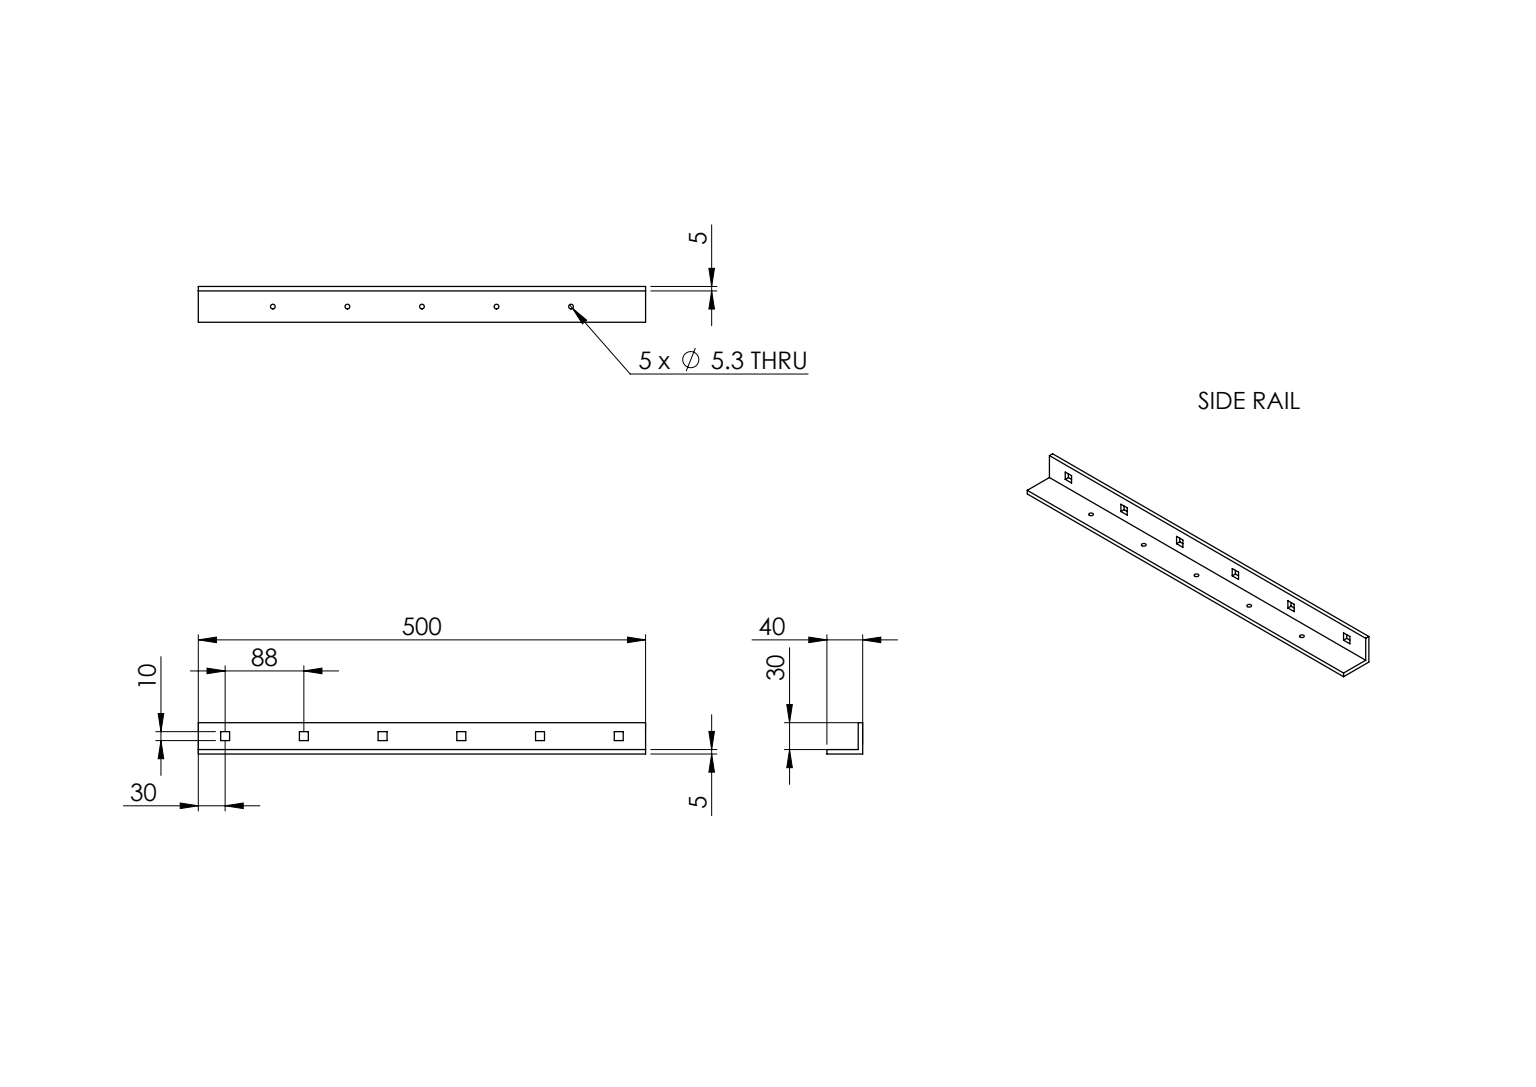
ISO-10303-21;
HEADER;
FILE_DESCRIPTION (('STEP AP214'),
    '1' );
FILE_NAME ('side rail.step',
    '2026-10-24T11:01:53',
    ( '' ),
    ( '' ),
    'SwSTEP 2.0',
    'SolidWorks 2026',
    '' );
FILE_SCHEMA (( 'AUTOMOTIVE_DESIGN' ));
ENDSEC;

DATA;
#13=PRODUCT_DEFINITION_FORMATION_WITH_SPECIFIED_SOURCE ( 'ANY', '', #8583, .NOT_KNOWN. ) ;
#18=CARTESIAN_POINT ( 'NONE',  ( 386.6666666666666288, -15.00000000000000000, 165.1500000000000625 ) ) ;
#24=VERTEX_POINT ( 'NONE', #6412 ) ;
#26=CARTESIAN_POINT ( 'NONE',  ( -30.00000000000000000, 15.00000000000000000, 145.0000000000000284 ) ) ;
#31=CARTESIAN_POINT ( 'NONE',  ( -4.999999999999998224, -4.999999999999998224, 145.0000000000000284 ) ) ;
#46=AXIS2_PLACEMENT_3D ( 'NONE', #70, #7390, #6602 ) ;
#48=VECTOR ( 'NONE', #1988, 1000.000000000000000 ) ;
#54=VERTEX_POINT ( 'NONE', #1769 ) ;
#58=VERTEX_POINT ( 'NONE', #5981 ) ;
#60=EDGE_CURVE ( 'NONE', #24, #4191, #63, .T. ) ;
#63=LINE ( 'NONE', #5464, #2595 ) ;
#67=EDGE_CURVE ( 'NONE', #3923, #3144, #6728, .T. ) ;
#70=CARTESIAN_POINT ( 'NONE',  ( 219.9999999999999716, -14.99999999999999822, 162.5000000000000853 ) ) ;
#87=ADVANCED_FACE ( 'NONE', ( #7344 ), #1423, .F. ) ;
#111=AXIS2_PLACEMENT_3D ( 'NONE', #1042, #3694, #1743 ) ;
#117=ORIENTED_EDGE ( 'NONE', *, *, #2503, .F. ) ;
#124=ORIENTED_EDGE ( 'NONE', *, *, #3492, .T. ) ;
#125=LINE ( 'NONE', #5958, #4603 ) ;
#149=CARTESIAN_POINT ( 'NONE',  ( -30.00000000000002842, -15.00000000000000000, 180.0000000000000284 ) ) ;
#156=VECTOR ( 'NONE', #5813, 1000.000000000000000 ) ;
#162=DIRECTION ( 'NONE',  ( -0.000000000000000000, -0.000000000000000000, 1.000000000000000000 ) ) ;
#167=ADVANCED_FACE ( 'NONE', ( #3513 ), #4000, .F. ) ;
#169=EDGE_LOOP ( 'NONE', ( #5952, #1913, #7757, #4086 ) ) ;
#170=DIRECTION ( 'NONE',  ( -1.000000000000000000, 0.000000000000000000, -0.000000000000000000 ) ) ;
#174=DIRECTION ( 'NONE',  ( 0.000000000000000000, -1.000000000000000000, 0.000000000000000000 ) ) ;
#182=CARTESIAN_POINT ( 'NONE',  ( 269.0000000000000000, -4.999999999999998224, 145.0000000000000284 ) ) ;
#186=VERTEX_POINT ( 'NONE', #5337 ) ;
#190=ORIENTED_EDGE ( 'NONE', *, *, #4626, .T. ) ;
#201=EDGE_CURVE ( 'NONE', #7722, #4892, #6771, .T. ) ;
#202=EDGE_CURVE ( 'NONE', #3923, #6024, #3423, .T. ) ;
#203=LINE ( 'NONE', #2266, #5375 ) ;
#208=ORIENTED_EDGE ( 'NONE', *, *, #6764, .T. ) ;
#220=AXIS2_PLACEMENT_3D ( 'NONE', #6944, #7654, #6292 ) ;
#234=EDGE_CURVE ( 'NONE', #3505, #4164, #2178, .T. ) ;
#238=VERTEX_POINT ( 'NONE', #4948 ) ;
#241=DIRECTION ( 'NONE',  ( 0.000000000000000000, 0.000000000000000000, 1.000000000000000000 ) ) ;
#244=FACE_OUTER_BOUND ( 'NONE', #4831, .T. ) ;
#245=LINE ( 'NONE', #4910, #2842 ) ;
#249=EDGE_CURVE ( 'NONE', #7704, #6568, #408, .T. ) ;
#254=ORIENTED_EDGE ( 'NONE', *, *, #6075, .T. ) ;
#255=DIRECTION ( 'NONE',  ( 0.000000000000000000, -1.000000000000000000, 0.000000000000000000 ) ) ;
#259=DIRECTION ( 'NONE',  ( 0.000000000000000000, 0.000000000000000000, 1.000000000000000000 ) ) ;
#263=VECTOR ( 'NONE', #6923, 1000.000000000000000 ) ;
#287=PLANE ( 'NONE',  #7700 ) ;
#289=CARTESIAN_POINT ( 'NONE',  ( 219.9999999999999716, -20.00000000000000000, 165.1500000000000625 ) ) ;
#298=DIRECTION ( 'NONE',  ( 0.000000000000000000, 0.000000000000000000, 1.000000000000000000 ) ) ;
#309=DIRECTION ( 'NONE',  ( 0.000000000000000000, 0.000000000000000000, 1.000000000000000000 ) ) ;
#318=ORIENTED_EDGE ( 'NONE', *, *, #3170, .T. ) ;
#324=DIRECTION ( 'NONE',  ( -0.000000000000000000, -0.000000000000000000, -1.000000000000000000 ) ) ;
#331=AXIS2_PLACEMENT_3D ( 'NONE', #650, #3395, #2654 ) ;
#333=CARTESIAN_POINT ( 'NONE',  ( 170.9999999999999716, 5.000000000000001776, 140.0000000000000000 ) ) ;
#347=ORIENTED_EDGE ( 'NONE', *, *, #4193, .T. ) ;
#361=ADVANCED_FACE ( 'NONE', ( #4903 ), #2861, .F. ) ;
#363=EDGE_CURVE ( 'NONE', #6062, #5755, #7748, .T. ) ;
#375=ORIENTED_EDGE ( 'NONE', *, *, #4660, .F. ) ;
#386=ORIENTED_EDGE ( 'NONE', *, *, #234, .T. ) ;
#388=LINE ( 'NONE', #2410, #2981 ) ;
#406=AXIS2_PLACEMENT_3D ( 'NONE', #5690, #1942, #2315 ) ;
#407=ORIENTED_EDGE ( 'NONE', *, *, #3455, .T. ) ;
#408=LINE ( 'NONE', #3556, #5504 ) ;
#413=ORIENTED_EDGE ( 'NONE', *, *, #6908, .F. ) ;
#416=SURFACE_STYLE_FILL_AREA ( #6943 ) ;
#427=CARTESIAN_POINT ( 'NONE',  ( 357.0000000000000000, -4.999999999999998224, 145.0000000000000284 ) ) ;
#429=ORIENTED_EDGE ( 'NONE', *, *, #1847, .T. ) ;
#431=DIRECTION ( 'NONE',  ( -1.734723475976807341E-16, 1.000000000000000000, 0.000000000000000000 ) ) ;
#433=DIRECTION ( 'NONE',  ( 0.000000000000000000, 0.000000000000000000, 1.000000000000000000 ) ) ;
#445=EDGE_CURVE ( 'NONE', #1439, #7609, #7238, .T. ) ;
#446=DIRECTION ( 'NONE',  ( 0.000000000000000000, 0.000000000000000000, 1.000000000000000000 ) ) ;
#448=ORIENTED_EDGE ( 'NONE', *, *, #1374, .T. ) ;
#464=DIRECTION ( 'NONE',  ( 0.000000000000000000, 0.000000000000000000, 1.000000000000000000 ) ) ;
#466=EDGE_LOOP ( 'NONE', ( #1944, #2418, #2156, #4919 ) ) ;
#472=APPLICATION_CONTEXT ( 'automotive_design' ) ;
#473=CARTESIAN_POINT ( 'NONE',  ( -30.00000000000002842, -20.00000000000000000, 180.0000000000000284 ) ) ;
#495=CARTESIAN_POINT ( 'NONE',  ( 136.6666666666666288, -14.99999999999999822, 162.5000000000000853 ) ) ;
#503=AXIS2_PLACEMENT_3D ( 'NONE', #3389, #7471, #6027 ) ;
#516=CIRCLE ( 'NONE', #3995, 2.649999999999985700 ) ;
#517=VECTOR ( 'NONE', #7391, 1000.000000000000000 ) ;
#522=CARTESIAN_POINT ( 'NONE',  ( 444.9999999999999432, -4.999999999999998224, 139.9990000000000236 ) ) ;
#524=CYLINDRICAL_SURFACE ( 'NONE', #783, 2.649999999999985700 ) ;
#527=ORIENTED_EDGE ( 'NONE', *, *, #5024, .F. ) ;
#539=AXIS2_PLACEMENT_3D ( 'NONE', #8100, #4108, #804 ) ;
#540=FACE_OUTER_BOUND ( 'NONE', #466, .T. ) ;
#545=CARTESIAN_POINT ( 'NONE',  ( 347.0000000000000000, 5.000000000000001776, 145.0000000000000284 ) ) ;
#547=DIRECTION ( 'NONE',  ( 0.000000000000000000, -1.000000000000000000, 0.000000000000000000 ) ) ;
#551=EDGE_CURVE ( 'NONE', #2756, #4735, #3107, .T. ) ;
#553=CARTESIAN_POINT ( 'NONE',  ( 259.0000000000000000, -4.999999999999998224, 140.0000000000000000 ) ) ;
#575=CARTESIAN_POINT ( 'NONE',  ( -30.00000000000002842, -20.00000000000000000, 180.0000000000000284 ) ) ;
#578=EDGE_CURVE ( 'NONE', #4191, #4735, #5829, .T. ) ;
#580=EDGE_CURVE ( 'NONE', #8517, #6781, #7849, .T. ) ;
#581=STYLED_ITEM('',(#8650),#4654);
#592=AXIS2_PLACEMENT_3D ( 'NONE', #1582, #4234, #309 ) ;
#594=AXIS2_PLACEMENT_3D ( 'NONE', #3123, #464, #5764 ) ;
#601=FACE_BOUND ( 'NONE', #6016, .T. ) ;
#603=VECTOR ( 'NONE', #2035, 1000.000000000000000 ) ;
#604=ORIENTED_EDGE ( 'NONE', *, *, #7855, .F. ) ;
#606=FACE_OUTER_BOUND ( 'NONE', #8585, .T. ) ;
#609=FACE_OUTER_BOUND ( 'NONE', #8309, .T. ) ;
#610=DIRECTION ( 'NONE',  ( 0.000000000000000000, -1.000000000000000000, 0.000000000000000000 ) ) ;
#611=ORIENTED_EDGE ( 'NONE', *, *, #6429, .F. ) ;
#616=VECTOR ( 'NONE', #2532, 1000.000000000000000 ) ;
#640=ORIENTED_EDGE ( 'NONE', *, *, #7790, .T. ) ;
#641=CARTESIAN_POINT ( 'NONE',  ( 444.9999999999999432, 5.000000000000000000, 145.0000000000000284 ) ) ;
#650=CARTESIAN_POINT ( 'NONE',  ( 82.99999999999998579, -4.999999999999998224, 139.9990000000000236 ) ) ;
#655=FACE_OUTER_BOUND ( 'NONE', #4653, .T. ) ;
#656=EDGE_LOOP ( 'NONE', ( #7632, #980, #7793, #6433 ) ) ;
#662=DIRECTION ( 'NONE',  ( -0.000000000000000000, 1.000000000000000000, -0.000000000000000000 ) ) ;
#667=CARTESIAN_POINT ( 'NONE',  ( 434.9999999999999432, 5.000000000000001776, 140.0000000000000000 ) ) ;
#673=DIRECTION ( 'NONE',  ( -0.000000000000000000, -0.000000000000000000, 1.000000000000000000 ) ) ;
#675=ORIENTED_EDGE ( 'NONE', *, *, #4538, .T. ) ;
#679=CARTESIAN_POINT ( 'NONE',  ( 386.6666666666666288, -20.00000000000000000, 159.8500000000001080 ) ) ;
#680=LINE ( 'NONE', #6020, #603 ) ;
#681=EDGE_CURVE ( 'NONE', #54, #5626, #751, .T. ) ;
#691=CARTESIAN_POINT ( 'NONE',  ( 259.0000000000000000, -4.999999999999998224, 145.0000000000000284 ) ) ;
#692=DIRECTION ( 'NONE',  ( 0.000000000000000000, 0.000000000000000000, 1.000000000000000000 ) ) ;
#694=DIRECTION ( 'NONE',  ( 1.000000000000000000, 1.734723475976807587E-16, 0.000000000000000000 ) ) ;
#698=ORIENTED_EDGE ( 'NONE', *, *, #7696, .T. ) ;
#705=DIRECTION ( 'NONE',  ( 1.000000000000000000, 0.000000000000000000, 0.000000000000000000 ) ) ;
#706=EDGE_CURVE ( 'NONE', #6409, #7056, #2096, .T. ) ;
#715=EDGE_LOOP ( 'NONE', ( #5309, #6953, #3557, #6643 ) ) ;
#716=VERTEX_POINT ( 'NONE', #3406 ) ;
#722=EDGE_LOOP ( 'NONE', ( #7433, #7623, #8054, #2319 ) ) ;
#729=DIRECTION ( 'NONE',  ( -0.000000000000000000, 1.000000000000000000, -0.000000000000000000 ) ) ;
#730=VERTEX_POINT ( 'NONE', #3974 ) ;
#733=DIRECTION ( 'NONE',  ( 0.000000000000000000, -1.000000000000000000, 0.000000000000000000 ) ) ;
#734=DIRECTION ( 'NONE',  ( 1.000000000000000000, 1.734723475976807587E-16, 0.000000000000000000 ) ) ;
#740=VECTOR ( 'NONE', #3211, 1000.000000000000000 ) ;
#749=VECTOR ( 'NONE', #5021, 1000.000000000000000 ) ;
#751=LINE ( 'NONE', #3447, #4670 ) ;
#753=ADVANCED_FACE ( 'NONE', ( #4656 ), #3358, .F. ) ;
#763=CARTESIAN_POINT ( 'NONE',  ( -30.00000000000000000, 15.00000000000000000, 145.0000000000000284 ) ) ;
#780=CARTESIAN_POINT ( 'NONE',  ( 434.9999999999999432, -4.999999999999998224, 145.0000000000000284 ) ) ;
#783=AXIS2_PLACEMENT_3D ( 'NONE', #5091, #5820, #5173 ) ;
#785=DIRECTION ( 'NONE',  ( 0.000000000000000000, 1.000000000000000000, 0.000000000000000000 ) ) ;
#786=ORIENTED_EDGE ( 'NONE', *, *, #578, .T. ) ;
#796=DIRECTION ( 'NONE',  ( -1.000000000000000000, 0.000000000000000000, 0.000000000000000000 ) ) ;
#804=DIRECTION ( 'NONE',  ( 0.000000000000000000, 0.000000000000000000, 1.000000000000000000 ) ) ;
#809=DIRECTION ( 'NONE',  ( 0.000000000000000000, 0.000000000000000000, 1.000000000000000000 ) ) ;
#819=VERTEX_POINT ( 'NONE', #4271 ) ;
#837=CARTESIAN_POINT ( 'NONE',  ( 347.0000000000000000, -4.999999999999998224, 145.0000000000000284 ) ) ;
#841=EDGE_CURVE ( 'NONE', #58, #2735, #4314, .T. ) ;
#849=EDGE_CURVE ( 'NONE', #874, #3144, #1486, .T. ) ;
#855=ORIENTED_EDGE ( 'NONE', *, *, #4193, .F. ) ;
#859=DIRECTION ( 'NONE',  ( -0.000000000000000000, 1.000000000000000000, -0.000000000000000000 ) ) ;
#861=ORIENTED_EDGE ( 'NONE', *, *, #3272, .T. ) ;
#874=VERTEX_POINT ( 'NONE', #6131 ) ;
#877=FACE_OUTER_BOUND ( 'NONE', #3003, .T. ) ;
#898=VECTOR ( 'NONE', #7582, 1000.000000000000000 ) ;
#902=DIRECTION ( 'NONE',  ( 0.000000000000000000, -0.000000000000000000, -1.000000000000000000 ) ) ;
#905=DIRECTION ( 'NONE',  ( 0.000000000000000000, 0.000000000000000000, -1.000000000000000000 ) ) ;
#911=FACE_OUTER_BOUND ( 'NONE', #8041, .T. ) ;
#920=CARTESIAN_POINT ( 'NONE',  ( 347.0000000000000000, -4.999999999999998224, 139.9990000000000236 ) ) ;
#925=FACE_BOUND ( 'NONE', #8290, .T. ) ;
#928=CARTESIAN_POINT ( 'NONE',  ( 470.0000000000000000, 15.00000000000000000, 140.0000000000000000 ) ) ;
#951=VERTEX_POINT ( 'NONE', #3223 ) ;
#955=LINE ( 'NONE', #3606, #3821 ) ;
#957=CARTESIAN_POINT ( 'NONE',  ( 219.9999999999999716, -20.00000000000000000, 162.5000000000000853 ) ) ;
#968=LINE ( 'NONE', #7447, #1506 ) ;
#970=PLANE ( 'NONE',  #4855 ) ;
#972=CARTESIAN_POINT ( 'NONE',  ( -30.00000000000002842, -20.00000000000000000, 180.0000000000000284 ) ) ;
#978=DIRECTION ( 'NONE',  ( 0.000000000000000000, 1.000000000000000000, 0.000000000000000000 ) ) ;
#979=ORIENTED_EDGE ( 'NONE', *, *, #3323, .F. ) ;
#980=ORIENTED_EDGE ( 'NONE', *, *, #7467, .T. ) ;
#984=ADVANCED_FACE ( 'NONE', ( #1052 ), #524, .F. ) ;
#986=ADVANCED_FACE ( 'NONE', ( #8495 ), #7673, .F. ) ;
#991=ORIENTED_EDGE ( 'NONE', *, *, #2182, .F. ) ;
#993=DIRECTION ( 'NONE',  ( -1.000000000000000000, 0.000000000000000000, 0.000000000000000000 ) ) ;
#1010=ADVANCED_FACE ( 'NONE', ( #6523 ), #8539, .F. ) ;
#1014=CARTESIAN_POINT ( 'NONE',  ( -4.999999999999998224, 5.000000000000001776, 139.9990000000000236 ) ) ;
#1023=ORIENTED_EDGE ( 'NONE', *, *, #5149, .T. ) ;
#1042=CARTESIAN_POINT ( 'NONE',  ( 386.6666666666666288, -15.00000000000000000, 162.5000000000000853 ) ) ;
#1048=ADVANCED_FACE ( 'NONE', ( #8418 ), #2454, .F. ) ;
#1050=DIRECTION ( 'NONE',  ( 0.000000000000000000, 0.000000000000000000, 1.000000000000000000 ) ) ;
#1052=FACE_OUTER_BOUND ( 'NONE', #5062, .T. ) ;
#1054=ORIENTED_EDGE ( 'NONE', *, *, #7248, .T. ) ;
#1055=DIRECTION ( 'NONE',  ( -1.000000000000000000, 0.000000000000000000, 0.000000000000000000 ) ) ;
#1067=LINE ( 'NONE', #8387, #5879 ) ;
#1078=ORIENTED_EDGE ( 'NONE', *, *, #5149, .F. ) ;
#1084=CARTESIAN_POINT ( 'NONE',  ( 347.0000000000000000, 5.000000000000001776, 145.0000000000000284 ) ) ;
#1092=CARTESIAN_POINT ( 'NONE',  ( -4.999999999999998224, 5.000000000000001776, 145.0000000000000284 ) ) ;
#1120=AXIS2_PLACEMENT_3D ( 'NONE', #2318, #4961, #4307 ) ;
#1123=VERTEX_POINT ( 'NONE', #2089 ) ;
#1125=DIRECTION ( 'NONE',  ( 1.000000000000000000, 0.000000000000000000, 0.000000000000000000 ) ) ;
#1126=FACE_OUTER_BOUND ( 'NONE', #2316, .T. ) ;
#1127=ORIENTED_EDGE ( 'NONE', *, *, #3594, .F. ) ;
#1129=ADVANCED_FACE ( 'NONE', ( #609 ), #3265, .F. ) ;
#1145=CARTESIAN_POINT ( 'NONE',  ( 269.0000000000000000, -4.999999999999998224, 145.0000000000000284 ) ) ;
#1149=EDGE_CURVE ( 'NONE', #3461, #2983, #5389, .T. ) ;
#1152=ADVANCED_FACE ( 'NONE', ( #3482 ), #8277, .T. ) ;
#1153=VECTOR ( 'NONE', #1857, 1000.000000000000000 ) ;
#1185=ORIENTED_EDGE ( 'NONE', *, *, #201, .F. ) ;
#1192=DIRECTION ( 'NONE',  ( 0.000000000000000000, 1.000000000000000000, 0.000000000000000000 ) ) ;
#1195=AXIS2_PLACEMENT_3D ( 'NONE', #7262, #694, #2743 ) ;
#1203=AXIS2_PLACEMENT_3D ( 'NONE', #5420, #8139, #5288 ) ;
#1204=ORIENTED_EDGE ( 'NONE', *, *, #4975, .T. ) ;
#1208=FACE_OUTER_BOUND ( 'NONE', #8313, .T. ) ;
#1210=CARTESIAN_POINT ( 'NONE',  ( 434.9999999999999432, -4.999999999999998224, 139.9990000000000236 ) ) ;
#1212=DIRECTION ( 'NONE',  ( -1.000000000000000000, 1.734723475976807341E-16, -0.000000000000000000 ) ) ;
#1213=EDGE_CURVE ( 'NONE', #730, #716, #6215, .T. ) ;
#1223=VECTOR ( 'NONE', #3407, 1000.000000000000000 ) ;
#1228=DIRECTION ( 'NONE',  ( -0.000000000000000000, 1.000000000000000000, -0.000000000000000000 ) ) ;
#1236=LINE ( 'NONE', #1279, #1910 ) ;
#1244=EDGE_CURVE ( 'NONE', #238, #4249, #5603, .T. ) ;
#1248=VERTEX_POINT ( 'NONE', #6169 ) ;
#1257=DIRECTION ( 'NONE',  ( 0.000000000000000000, -0.000000000000000000, -1.000000000000000000 ) ) ;
#1263=EDGE_CURVE ( 'NONE', #1874, #8118, #8146, .T. ) ;
#1276=EDGE_CURVE ( 'NONE', #2983, #951, #203, .T. ) ;
#1279=CARTESIAN_POINT ( 'NONE',  ( 82.99999999999998579, -4.999999999999998224, 145.0000000000000284 ) ) ;
#1281=VECTOR ( 'NONE', #1939, 1000.000000000000000 ) ;
#1286=CARTESIAN_POINT ( 'NONE',  ( 219.9999999999999716, -14.99999999999999822, 159.8500000000001080 ) ) ;
#1294=CARTESIAN_POINT ( 'NONE',  ( 0.000000000000000000, 0.000000000000000000, 145.0000000000000284 ) ) ;
#1313=CARTESIAN_POINT ( 'NONE',  ( 259.0000000000000000, -4.999999999999998224, 145.0000000000000284 ) ) ;
#1316=CARTESIAN_POINT ( 'NONE',  ( 181.0000000000000000, 5.000000000000000000, 145.0000000000000284 ) ) ;
#1318=LINE ( 'NONE', #1360, #3234 ) ;
#1320=CARTESIAN_POINT ( 'NONE',  ( 303.3333333333333144, -20.00000000000000000, 162.5000000000000853 ) ) ;
#1331=ORIENTED_EDGE ( 'NONE', *, *, #6988, .T. ) ;
#1335=CARTESIAN_POINT ( 'NONE',  ( 219.9999999999999716, -15.00000000000000000, 162.5000000000000853 ) ) ;
#1340=PLANE ( 'NONE',  #6168 ) ;
#1341=ADVANCED_FACE ( 'NONE', ( #1126 ), #3869, .F. ) ;
#1360=CARTESIAN_POINT ( 'NONE',  ( 444.9999999999999432, -4.999999999999998224, 140.0000000000000000 ) ) ;
#1362=CARTESIAN_POINT ( 'NONE',  ( 82.99999999999998579, -4.999999999999998224, 140.0000000000000000 ) ) ;
#1363=LINE ( 'NONE', #3985, #3019 ) ;
#1374=EDGE_CURVE ( 'NONE', #1123, #951, #3693, .T. ) ;
#1375=EDGE_CURVE ( 'NONE', #4726, #7555, #7127, .T. ) ;
#1377=DIRECTION ( 'NONE',  ( 1.000000000000000000, 0.000000000000000000, 0.000000000000000000 ) ) ;
#1386=ORIENTED_EDGE ( 'NONE', *, *, #1213, .T. ) ;
#1390=DIRECTION ( 'NONE',  ( 1.734723475976807587E-16, 1.000000000000000000, 0.000000000000000000 ) ) ;
#1406=CARTESIAN_POINT ( 'NONE',  ( 470.0000000000000000, 15.00000000000000000, 140.0000000000000000 ) ) ;
#1413=CARTESIAN_POINT ( 'NONE',  ( 434.9999999999999432, 5.000000000000001776, 139.9990000000000236 ) ) ;
#1421=ORIENTED_EDGE ( 'NONE', *, *, #7067, .T. ) ;
#1423=PLANE ( 'NONE',  #5781 ) ;
#1427=VECTOR ( 'NONE', #7633, 1000.000000000000000 ) ;
#1436=ORIENTED_EDGE ( 'NONE', *, *, #4897, .F. ) ;
#1439=VERTEX_POINT ( 'NONE', #2688 ) ;
#1441=CARTESIAN_POINT ( 'NONE',  ( 170.9999999999999716, 5.000000000000001776, 145.0000000000000284 ) ) ;
#1442=AXIS2_PLACEMENT_3D ( 'NONE', #2110, #4768, #809 ) ;
#1445=FACE_OUTER_BOUND ( 'NONE', #6630, .T. ) ;
#1449=LINE ( 'NONE', #4887, #2264 ) ;
#1456=EDGE_CURVE ( 'NONE', #7186, #4028, #5849, .T. ) ;
#1465=DIRECTION ( 'NONE',  ( -1.000000000000000000, 0.000000000000000000, 0.000000000000000000 ) ) ;
#1466=DIRECTION ( 'NONE',  ( 0.000000000000000000, -1.000000000000000000, 0.000000000000000000 ) ) ;
#1472=CARTESIAN_POINT ( 'NONE',  ( 434.9999999999999432, -4.999999999999998224, 140.0000000000000000 ) ) ;
#1475=ORIENTED_EDGE ( 'NONE', *, *, #3348, .T. ) ;
#1486=CIRCLE ( 'NONE', #7458, 2.649999999999985700 ) ;
#1492=CARTESIAN_POINT ( 'NONE',  ( 0.000000000000000000, 0.000000000000000000, 140.0000000000000000 ) ) ;
#1506=VECTOR ( 'NONE', #6180, 1000.000000000000000 ) ;
#1507=ORIENTED_EDGE ( 'NONE', *, *, #6503, .T. ) ;
#1519=DIRECTION ( 'NONE',  ( 0.000000000000000000, 1.000000000000000000, 0.000000000000000000 ) ) ;
#1520=CARTESIAN_POINT ( 'NONE',  ( -30.00000000000000000, 15.00000000000000000, 145.0000000000000284 ) ) ;
#1531=CARTESIAN_POINT ( 'NONE',  ( 5.000000000000001776, -4.999999999999998224, 145.0000000000000284 ) ) ;
#1534=ORIENTED_EDGE ( 'NONE', *, *, #3805, .T. ) ;
#1545=ORIENTED_EDGE ( 'NONE', *, *, #5785, .T. ) ;
#1547=CARTESIAN_POINT ( 'NONE',  ( 470.0000000000000000, -20.00000000000000000, 180.0000000000000284 ) ) ;
#1549=VERTEX_POINT ( 'NONE', #5244 ) ;
#1559=CARTESIAN_POINT ( 'NONE',  ( 470.0000000000000000, 15.00000000000000000, 145.0000000000000284 ) ) ;
#1571=CARTESIAN_POINT ( 'NONE',  ( 357.0000000000000000, -4.999999999999998224, 140.0000000000000000 ) ) ;
#1575=EDGE_CURVE ( 'NONE', #4726, #2056, #1912, .T. ) ;
#1581=LINE ( 'NONE', #6883, #6243 ) ;
#1582=CARTESIAN_POINT ( 'NONE',  ( 219.9999999999999716, -20.00000000000000000, 162.5000000000000853 ) ) ;
#1621=ORIENTED_EDGE ( 'NONE', *, *, #4246, .T. ) ;
#1622=DIRECTION ( 'NONE',  ( 0.000000000000000000, 0.000000000000000000, -1.000000000000000000 ) ) ;
#1625=CARTESIAN_POINT ( 'NONE',  ( -4.999999999999998224, 5.000000000000001776, 140.0000000000000000 ) ) ;
#1631=DIRECTION ( 'NONE',  ( -0.000000000000000000, -0.000000000000000000, 1.000000000000000000 ) ) ;
#1638=LINE ( 'NONE', #1727, #5607 ) ;
#1640=ORIENTED_EDGE ( 'NONE', *, *, #5969, .F. ) ;
#1645=CARTESIAN_POINT ( 'NONE',  ( -4.999999999999998224, -4.999999999999998224, 139.9990000000000236 ) ) ;
#1654=EDGE_CURVE ( 'NONE', #3461, #1123, #2900, .T. ) ;
#1656=CARTESIAN_POINT ( 'NONE',  ( 386.6666666666666288, -14.99999999999999822, 165.1500000000000625 ) ) ;
#1659=DIRECTION ( 'NONE',  ( -1.000000000000000000, 1.734723475976807341E-16, -0.000000000000000000 ) ) ;
#1680=ORIENTED_EDGE ( 'NONE', *, *, #578, .F. ) ;
#1682=LINE ( 'NONE', #3073, #8263 ) ;
#1699=ADVANCED_FACE ( 'NONE', ( #2773 ), #2116, .F. ) ;
#1707=ORIENTED_EDGE ( 'NONE', *, *, #3455, .F. ) ;
#1710=CARTESIAN_POINT ( 'NONE',  ( 0.000000000000000000, -15.00000000000000000, 0.000000000000000000 ) ) ;
#1725=ORIENTED_EDGE ( 'NONE', *, *, #202, .T. ) ;
#1727=CARTESIAN_POINT ( 'NONE',  ( 5.000000000000000000, 5.000000000000000000, 139.9990000000000236 ) ) ;
#1736=ORIENTED_EDGE ( 'NONE', *, *, #7668, .T. ) ;
#1737=ORIENTED_EDGE ( 'NONE', *, *, #6829, .F. ) ;
#1738=VECTOR ( 'NONE', #431, 1000.000000000000000 ) ;
#1739=CARTESIAN_POINT ( 'NONE',  ( 347.0000000000000000, 5.000000000000001776, 139.9990000000000236 ) ) ;
#1743=DIRECTION ( 'NONE',  ( 0.000000000000000000, 0.000000000000000000, 1.000000000000000000 ) ) ;
#1750=DIRECTION ( 'NONE',  ( -0.000000000000000000, -1.000000000000000000, -0.000000000000000000 ) ) ;
#1764=CARTESIAN_POINT ( 'NONE',  ( 136.6666666666666288, -20.00000000000000000, 162.5000000000000853 ) ) ;
#1769=CARTESIAN_POINT ( 'NONE',  ( 53.33333333333330017, -20.00000000000000000, 159.8500000000001080 ) ) ;
#1778=PRESENTATION_STYLE_ASSIGNMENT (( #7741 ) ) ;
#1797=DIRECTION ( 'NONE',  ( -0.000000000000000000, 1.000000000000000000, -0.000000000000000000 ) ) ;
#1799=ORIENTED_EDGE ( 'NONE', *, *, #5024, .T. ) ;
#1802=DIRECTION ( 'NONE',  ( 0.000000000000000000, 0.000000000000000000, 1.000000000000000000 ) ) ;
#1808=AXIS2_PLACEMENT_3D ( 'NONE', #2841, #4317, #4797 ) ;
#1821=VECTOR ( 'NONE', #1228, 1000.000000000000000 ) ;
#1847=EDGE_CURVE ( 'NONE', #7056, #2677, #5115, .T. ) ;
#1854=AXIS2_PLACEMENT_3D ( 'NONE', #972, #2843, #2193 ) ;
#1857=DIRECTION ( 'NONE',  ( -0.000000000000000000, -0.000000000000000000, 1.000000000000000000 ) ) ;
#1874=VERTEX_POINT ( 'NONE', #4583 ) ;
#1879=EDGE_LOOP ( 'NONE', ( #4286, #2247, #979, #604 ) ) ;
#1880=DIRECTION ( 'NONE',  ( -0.000000000000000000, -0.000000000000000000, 1.000000000000000000 ) ) ;
#1881=CARTESIAN_POINT ( 'NONE',  ( -4.999999999999998224, -4.999999999999998224, 139.9990000000000236 ) ) ;
#1883=DIRECTION ( 'NONE',  ( 1.000000000000000000, 1.734723475976807587E-16, 0.000000000000000000 ) ) ;
#1892=EDGE_CURVE ( 'NONE', #7220, #7011, #1236, .T. ) ;
#1894=DIRECTION ( 'NONE',  ( 0.000000000000000000, 0.000000000000000000, 1.000000000000000000 ) ) ;
#1896=DIRECTION ( 'NONE',  ( 1.734723475976807587E-16, 1.000000000000000000, 0.000000000000000000 ) ) ;
#1907=VERTEX_POINT ( 'NONE', #6666 ) ;
#1910=VECTOR ( 'NONE', #4669, 1000.000000000000000 ) ;
#1911=VECTOR ( 'NONE', #2188, 1000.000000000000000 ) ;
#1912=LINE ( 'NONE', #4549, #3150 ) ;
#1913=ORIENTED_EDGE ( 'NONE', *, *, #4759, .T. ) ;
#1926=PLANE ( 'NONE',  #5252 ) ;
#1929=EDGE_LOOP ( 'NONE', ( #6294, #2936, #2091, #3597 ) ) ;
#1937=CARTESIAN_POINT ( 'NONE',  ( 82.99999999999998579, -4.999999999999998224, 145.0000000000000284 ) ) ;
#1939=DIRECTION ( 'NONE',  ( -0.000000000000000000, -1.000000000000000000, -0.000000000000000000 ) ) ;
#1940=CIRCLE ( 'NONE', #2504, 2.649999999999985700 ) ;
#1942=DIRECTION ( 'NONE',  ( -0.000000000000000000, 1.000000000000000000, -0.000000000000000000 ) ) ;
#1944=ORIENTED_EDGE ( 'NONE', *, *, #3170, .F. ) ;
#1949=EDGE_CURVE ( 'NONE', #24, #2756, #1363, .T. ) ;
#1950=LINE ( 'NONE', #6510, #740 ) ;
#1951=PRODUCT_DEFINITION_CONTEXT ( 'detailed design', #472, 'design' ) ;
#1979=DIRECTION ( 'NONE',  ( -0.000000000000000000, -0.000000000000000000, 1.000000000000000000 ) ) ;
#1988=DIRECTION ( 'NONE',  ( -1.000000000000000000, 1.734723475976807341E-16, -0.000000000000000000 ) ) ;
#1992=EDGE_CURVE ( 'NONE', #2774, #8517, #6758, .T. ) ;
#1997=DIRECTION ( 'NONE',  ( 0.000000000000000000, -1.000000000000000000, 0.000000000000000000 ) ) ;
#2002=EDGE_CURVE ( 'NONE', #2677, #3177, #3589, .T. ) ;
#2006=CARTESIAN_POINT ( 'NONE',  ( 259.0000000000000000, -4.999999999999998224, 140.0000000000000000 ) ) ;
#2007=PLANE ( 'NONE',  #4640 ) ;
#2011=DIRECTION ( 'NONE',  ( 0.000000000000000000, 0.000000000000000000, 1.000000000000000000 ) ) ;
#2025=EDGE_CURVE ( 'NONE', #4249, #2756, #8082, .T. ) ;
#2032=ORIENTED_EDGE ( 'NONE', *, *, #6244, .F. ) ;
#2035=DIRECTION ( 'NONE',  ( -0.000000000000000000, 1.000000000000000000, -0.000000000000000000 ) ) ;
#2046=ORIENTED_EDGE ( 'NONE', *, *, #5828, .T. ) ;
#2047=ORIENTED_EDGE ( 'NONE', *, *, #7067, .F. ) ;
#2055=CARTESIAN_POINT ( 'NONE',  ( 181.0000000000000000, 5.000000000000000000, 140.0000000000000000 ) ) ;
#2056=VERTEX_POINT ( 'NONE', #7457 ) ;
#2058=EDGE_LOOP ( 'NONE', ( #5168, #7419, #5067, #3478 ) ) ;
#2069=DIRECTION ( 'NONE',  ( 0.000000000000000000, 1.000000000000000000, 0.000000000000000000 ) ) ;
#2073=EDGE_LOOP ( 'NONE', ( #4749, #5157, #4998, #4326 ) ) ;
#2074=UNCERTAINTY_MEASURE_WITH_UNIT (LENGTH_MEASURE( 1.000000000000000082E-05 ), #6421, 'distance_accuracy_value', 'NONE');
#2077=DIRECTION ( 'NONE',  ( -1.000000000000000000, 1.734723475976807587E-16, 0.000000000000000000 ) ) ;
#2084=ORIENTED_EDGE ( 'NONE', *, *, #5522, .F. ) ;
#2087=DIRECTION ( 'NONE',  ( -1.000000000000000000, 0.000000000000000000, 0.000000000000000000 ) ) ;
#2089=CARTESIAN_POINT ( 'NONE',  ( 170.9999999999999716, -4.999999999999998224, 145.0000000000000284 ) ) ;
#2091=ORIENTED_EDGE ( 'NONE', *, *, #7723, .F. ) ;
#2093=ORIENTED_EDGE ( 'NONE', *, *, #6636, .F. ) ;
#2094=ORIENTED_EDGE ( 'NONE', *, *, #4865, .T. ) ;
#2096=LINE ( 'NONE', #4614, #4128 ) ;
#2110=CARTESIAN_POINT ( 'NONE',  ( 219.9999999999999716, -14.99999999999999822, 162.5000000000000853 ) ) ;
#2116=PLANE ( 'NONE',  #8301 ) ;
#2121=ORIENTED_EDGE ( 'NONE', *, *, #1992, .F. ) ;
#2125=DIRECTION ( 'NONE',  ( -1.000000000000000000, 1.734723475976807587E-16, 0.000000000000000000 ) ) ;
#2148=DIRECTION ( 'NONE',  ( -0.000000000000000000, 1.000000000000000000, -0.000000000000000000 ) ) ;
#2156=ORIENTED_EDGE ( 'NONE', *, *, #6669, .T. ) ;
#2158=EDGE_LOOP ( 'NONE', ( #7240, #5370, #4894, #5430 ) ) ;
#2160=PLANE ( 'NONE',  #7138 ) ;
#2162=CARTESIAN_POINT ( 'NONE',  ( 259.0000000000000000, -4.999999999999998224, 139.9990000000000236 ) ) ;
#2163=ORIENTED_EDGE ( 'NONE', *, *, #7799, .F. ) ;
#2172=DIRECTION ( 'NONE',  ( 1.000000000000000000, 0.000000000000000000, 0.000000000000000000 ) ) ;
#2177=EDGE_CURVE ( 'NONE', #2249, #1907, #8031, .T. ) ;
#2178=CIRCLE ( 'NONE', #220, 2.649999999999985700 ) ;
#2182=EDGE_CURVE ( 'NONE', #5694, #3602, #5625, .T. ) ;
#2188=DIRECTION ( 'NONE',  ( -1.734723475976807341E-16, 1.000000000000000000, 0.000000000000000000 ) ) ;
#2191=FACE_BOUND ( 'NONE', #7342, .T. ) ;
#2193=DIRECTION ( 'NONE',  ( 1.000000000000000000, 0.000000000000000000, 0.000000000000000000 ) ) ;
#2214=DIRECTION ( 'NONE',  ( 1.000000000000000000, 0.000000000000000000, 0.000000000000000000 ) ) ;
#2229=EDGE_CURVE ( 'NONE', #4164, #3505, #516, .T. ) ;
#2238=CARTESIAN_POINT ( 'NONE',  ( 93.00000000000000000, -4.999999999999998224, 140.0000000000000000 ) ) ;
#2247=ORIENTED_EDGE ( 'NONE', *, *, #1992, .T. ) ;
#2249=VERTEX_POINT ( 'NONE', #8594 ) ;
#2257=EDGE_LOOP ( 'NONE', ( #2935, #6507, #7530, #2667 ) ) ;
#2259=CARTESIAN_POINT ( 'NONE',  ( 303.3333333333333144, -20.00000000000000000, 159.8500000000001080 ) ) ;
#2260=VECTOR ( 'NONE', #7986, 1000.000000000000000 ) ;
#2264=VECTOR ( 'NONE', #8036, 1000.000000000000000 ) ;
#2266=CARTESIAN_POINT ( 'NONE',  ( 181.0000000000000000, -4.999999999999998224, 139.9990000000000236 ) ) ;
#2278=AXIS2_PLACEMENT_3D ( 'NONE', #5863, #6593, #2565 ) ;
#2283=LINE ( 'NONE', #4929, #263 ) ;
#2284=VECTOR ( 'NONE', #2214, 1000.000000000000000 ) ;
#2286=VECTOR ( 'NONE', #8261, 1000.000000000000000 ) ;
#2290=LINE ( 'NONE', #4934, #2510 ) ;
#2293=ORIENTED_EDGE ( 'NONE', *, *, #7855, .T. ) ;
#2311=EDGE_CURVE ( 'NONE', #716, #5369, #4748, .T. ) ;
#2315=DIRECTION ( 'NONE',  ( 0.000000000000000000, 0.000000000000000000, 1.000000000000000000 ) ) ;
#2316=EDGE_LOOP ( 'NONE', ( #7296, #407, #8302, #7762 ) ) ;
#2318=CARTESIAN_POINT ( 'NONE',  ( 357.0000000000000000, -4.999999999999998224, 139.9990000000000236 ) ) ;
#2319=ORIENTED_EDGE ( 'NONE', *, *, #6075, .F. ) ;
#2330=DIRECTION ( 'NONE',  ( -0.000000000000000000, -0.000000000000000000, -1.000000000000000000 ) ) ;
#2342=CARTESIAN_POINT ( 'NONE',  ( -30.00000000000002842, -15.00000000000000000, 145.0000000000000284 ) ) ;
#2353=EDGE_LOOP ( 'NONE', ( #3218, #4790, #5597, #7120 ) ) ;
#2363=CARTESIAN_POINT ( 'NONE',  ( 444.9999999999999432, -4.999999999999998224, 139.9990000000000236 ) ) ;
#2365=VECTOR ( 'NONE', #5347, 1000.000000000000000 ) ;
#2367=CARTESIAN_POINT ( 'NONE',  ( 357.0000000000000000, -4.999999999999998224, 139.9990000000000236 ) ) ;
#2368=ORIENTED_EDGE ( 'NONE', *, *, #2025, .F. ) ;
#2369=FACE_OUTER_BOUND ( 'NONE', #2058, .T. ) ;
#2371=VECTOR ( 'NONE', #1631, 1000.000000000000000 ) ;
#2372=DIRECTION ( 'NONE',  ( -0.000000000000000000, -0.000000000000000000, 1.000000000000000000 ) ) ;
#2375=EDGE_CURVE ( 'NONE', #238, #24, #4015, .T. ) ;
#2397=CARTESIAN_POINT ( 'NONE',  ( 470.0000000000000000, -20.00000000000000000, 180.0000000000000284 ) ) ;
#2400=DIRECTION ( 'NONE',  ( -0.000000000000000000, 1.000000000000000000, -0.000000000000000000 ) ) ;
#2404=CARTESIAN_POINT ( 'NONE',  ( 170.9999999999999716, 5.000000000000001776, 145.0000000000000284 ) ) ;
#2410=CARTESIAN_POINT ( 'NONE',  ( -4.999999999999998224, -4.999999999999998224, 145.0000000000000284 ) ) ;
#2418=ORIENTED_EDGE ( 'NONE', *, *, #6429, .T. ) ;
#2427=DIRECTION ( 'NONE',  ( -0.000000000000000000, -0.000000000000000000, 1.000000000000000000 ) ) ;
#2430=MECHANICAL_DESIGN_GEOMETRIC_PRESENTATION_REPRESENTATION('',(#4916),#2698);
#2439=ORIENTED_EDGE ( 'NONE', *, *, #5785, .F. ) ;
#2444=FACE_OUTER_BOUND ( 'NONE', #4566, .T. ) ;
#2445=CARTESIAN_POINT ( 'NONE',  ( 259.0000000000000000, -4.999999999999998224, 140.0000000000000000 ) ) ;
#2450=ORIENTED_EDGE ( 'NONE', *, *, #8409, .T. ) ;
#2451=VERTEX_POINT ( 'NONE', #4053 ) ;
#2454=PLANE ( 'NONE',  #1195 ) ;
#2455=ADVANCED_FACE ( 'NONE', ( #4615 ), #6615, .F. ) ;
#2477=EDGE_LOOP ( 'NONE', ( #1736, #6913, #190, #4003 ) ) ;
#2478=( NAMED_UNIT ( * ) PLANE_ANGLE_UNIT ( ) SI_UNIT ( $, .RADIAN. ) );
#2481=ORIENTED_EDGE ( 'NONE', *, *, #7318, .T. ) ;
#2486=VECTOR ( 'NONE', #5399, 1000.000000000000000 ) ;
#2503=EDGE_CURVE ( 'NONE', #2451, #3613, #968, .T. ) ;
#2504=AXIS2_PLACEMENT_3D ( 'NONE', #1320, #2069, #7371 ) ;
#2510=VECTOR ( 'NONE', #8253, 1000.000000000000000 ) ;
#2513=LINE ( 'NONE', #7988, #1153 ) ;
#2518=VECTOR ( 'NONE', #1659, 1000.000000000000000 ) ;
#2519=ORIENTED_EDGE ( 'NONE', *, *, #3228, .T. ) ;
#2528=ORIENTED_EDGE ( 'NONE', *, *, #2663, .F. ) ;
#2532=DIRECTION ( 'NONE',  ( -1.000000000000000000, 1.734723475976807341E-16, -0.000000000000000000 ) ) ;
#2560=ADVANCED_FACE ( 'NONE', ( #1445 ), #7585, .F. ) ;
#2565=DIRECTION ( 'NONE',  ( -1.000000000000000000, 1.734723475976807587E-16, 0.000000000000000000 ) ) ;
#2577=CARTESIAN_POINT ( 'NONE',  ( 53.33333333333330017, -15.00000000000000000, 162.5000000000000853 ) ) ;
#2589=DIRECTION ( 'NONE',  ( -0.000000000000000000, -0.000000000000000000, 1.000000000000000000 ) ) ;
#2595=VECTOR ( 'NONE', #7384, 1000.000000000000000 ) ;
#2599=ORIENTED_EDGE ( 'NONE', *, *, #6716, .T. ) ;
#2601=DIRECTION ( 'NONE',  ( -0.000000000000000000, 1.000000000000000000, -0.000000000000000000 ) ) ;
#2609=FACE_BOUND ( 'NONE', #2257, .T. ) ;
#2614=PRODUCT_DEFINITION ( 'UNKNOWN', '', #13, #1951 ) ;
#2619=CARTESIAN_POINT ( 'NONE',  ( 5.000000000000001776, -4.999999999999998224, 140.0000000000000000 ) ) ;
#2628=EDGE_CURVE ( 'NONE', #3075, #5045, #2922, .T. ) ;
#2630=ADVANCED_FACE ( 'NONE', ( #925, #3618, #4795, #6790, #4840, #7493 ), #5568, .T. ) ;
#2636=ORIENTED_EDGE ( 'NONE', *, *, #7800, .F. ) ;
#2637=SHAPE_REPRESENTATION_RELATIONSHIP ( 'NONE' , 'NONE' ,  #7993, #3452 ) ;
#2638=VERTEX_POINT ( 'NONE', #4358 ) ;
#2641=AXIS2_PLACEMENT_3D ( 'NONE', #3709, #1055, #4361 ) ;
#2650=FACE_OUTER_BOUND ( 'NONE', #5636, .T. ) ;
#2654=DIRECTION ( 'NONE',  ( 0.000000000000000000, -0.000000000000000000, -1.000000000000000000 ) ) ;
#2663=EDGE_CURVE ( 'NONE', #5369, #5286, #7802, .T. ) ;
#2667=ORIENTED_EDGE ( 'NONE', *, *, #1892, .F. ) ;
#2672=LINE ( 'NONE', #1092, #616 ) ;
#2677=VERTEX_POINT ( 'NONE', #7675 ) ;
#2685=PLANE ( 'NONE',  #2278 ) ;
#2688=CARTESIAN_POINT ( 'NONE',  ( 53.33333333333330017, -20.00000000000000000, 165.1500000000000625 ) ) ;
#2689=ORIENTED_EDGE ( 'NONE', *, *, #5886, .T. ) ;
#2691=CARTESIAN_POINT ( 'NONE',  ( 82.99999999999998579, -4.999999999999998224, 139.9990000000000236 ) ) ;
#2698=( GEOMETRIC_REPRESENTATION_CONTEXT ( 3 ) GLOBAL_UNCERTAINTY_ASSIGNED_CONTEXT ( ( #2074 ) ) GLOBAL_UNIT_ASSIGNED_CONTEXT ( ( #6421, #4250, #3288 ) ) REPRESENTATION_CONTEXT ( 'NONE', 'WORKASPACE' ) );
#2713=CARTESIAN_POINT ( 'NONE',  ( 434.9999999999999432, -4.999999999999998224, 139.9990000000000236 ) ) ;
#2727=FACE_OUTER_BOUND ( 'NONE', #5733, .T. ) ;
#2731=CARTESIAN_POINT ( 'NONE',  ( -30.00000000000002842, -20.00000000000000000, 140.0000000000000000 ) ) ;
#2735=VERTEX_POINT ( 'NONE', #3014 ) ;
#2736=ORIENTED_EDGE ( 'NONE', *, *, #6244, .T. ) ;
#2743=DIRECTION ( 'NONE',  ( -1.734723475976807587E-16, 1.000000000000000000, 0.000000000000000000 ) ) ;
#2750=ORIENTED_EDGE ( 'NONE', *, *, #551, .T. ) ;
#2756=VERTEX_POINT ( 'NONE', #7219 ) ;
#2758=ADVANCED_FACE ( 'NONE', ( #655 ), #1926, .F. ) ;
#2765=EDGE_LOOP ( 'NONE', ( #5019, #4745 ) ) ;
#2771=VECTOR ( 'NONE', #7329, 1000.000000000000000 ) ;
#2773=FACE_OUTER_BOUND ( 'NONE', #2353, .T. ) ;
#2774=VERTEX_POINT ( 'NONE', #3266 ) ;
#2777=AXIS2_PLACEMENT_3D ( 'NONE', #3153, #1192, #3849 ) ;
#2795=EDGE_LOOP ( 'NONE', ( #4476, #3760, #7438, #3041 ) ) ;
#2832=( GEOMETRIC_REPRESENTATION_CONTEXT ( 3 ) GLOBAL_UNCERTAINTY_ASSIGNED_CONTEXT ( ( #4675 ) ) GLOBAL_UNIT_ASSIGNED_CONTEXT ( ( #6248, #2478, #8350 ) ) REPRESENTATION_CONTEXT ( 'NONE', 'WORKASPACE' ) );
#2840=EDGE_LOOP ( 'NONE', ( #2121, #1707, #855, #7763 ) ) ;
#2841=CARTESIAN_POINT ( 'NONE',  ( 0.000000000000000000, -20.00000000000000000, 0.000000000000000000 ) ) ;
#2842=VECTOR ( 'NONE', #2125, 1000.000000000000000 ) ;
#2843=DIRECTION ( 'NONE',  ( -0.000000000000000000, 0.000000000000000000, 1.000000000000000000 ) ) ;
#2845=ADVANCED_FACE ( 'NONE', ( #7309 ), #6691, .F. ) ;
#2849=CARTESIAN_POINT ( 'NONE',  ( 444.9999999999999432, -4.999999999999998224, 145.0000000000000284 ) ) ;
#2853=ORIENTED_EDGE ( 'NONE', *, *, #8476, .T. ) ;
#2855=CARTESIAN_POINT ( 'NONE',  ( -4.999999999999998224, -4.999999999999998224, 140.0000000000000000 ) ) ;
#2861=PLANE ( 'NONE',  #2873 ) ;
#2865=EDGE_CURVE ( 'NONE', #1248, #58, #7924, .T. ) ;
#2866=CARTESIAN_POINT ( 'NONE',  ( -30.00000000000002842, -15.00000000000000000, 140.0000000000000000 ) ) ;
#2869=DIRECTION ( 'NONE',  ( -0.000000000000000000, -0.000000000000000000, 1.000000000000000000 ) ) ;
#2873=AXIS2_PLACEMENT_3D ( 'NONE', #1645, #4294, #7564 ) ;
#2875=VERTEX_POINT ( 'NONE', #2055 ) ;
#2877=DIRECTION ( 'NONE',  ( -0.000000000000000000, 1.000000000000000000, -0.000000000000000000 ) ) ;
#2880=CARTESIAN_POINT ( 'NONE',  ( 259.0000000000000000, -4.999999999999998224, 139.9990000000000236 ) ) ;
#2900=LINE ( 'NONE', #8178, #7452 ) ;
#2901=ORIENTED_EDGE ( 'NONE', *, *, #4626, .F. ) ;
#2902=CARTESIAN_POINT ( 'NONE',  ( 303.3333333333333144, -20.00000000000000000, 162.5000000000000853 ) ) ;
#2922=LINE ( 'NONE', #837, #8190 ) ;
#2925=FACE_OUTER_BOUND ( 'NONE', #4152, .T. ) ;
#2930=CARTESIAN_POINT ( 'NONE',  ( 470.0000000000000000, -20.00000000000000000, 140.0000000000000000 ) ) ;
#2935=ORIENTED_EDGE ( 'NONE', *, *, #8409, .F. ) ;
#2936=ORIENTED_EDGE ( 'NONE', *, *, #841, .T. ) ;
#2938=LINE ( 'NONE', #7775, #2286 ) ;
#2941=EDGE_LOOP ( 'NONE', ( #527, #4676, #2736, #2084 ) ) ;
#2946=EDGE_CURVE ( 'NONE', #7213, #3247, #3466, .T. ) ;
#2958=LINE ( 'NONE', #2404, #2518 ) ;
#2968=DIRECTION ( 'NONE',  ( -0.000000000000000000, 1.000000000000000000, -0.000000000000000000 ) ) ;
#2971=FACE_BOUND ( 'NONE', #2477, .T. ) ;
#2978=LINE ( 'NONE', #7638, #7500 ) ;
#2981=VECTOR ( 'NONE', #1750, 1000.000000000000000 ) ;
#2983=VERTEX_POINT ( 'NONE', #4218 ) ;
#2987=CARTESIAN_POINT ( 'NONE',  ( 53.33333333333330017, -14.99999999999999822, 165.1500000000000625 ) ) ;
#2988=AXIS2_PLACEMENT_3D ( 'NONE', #8239, #2877, #298 ) ;
#2996=DIRECTION ( 'NONE',  ( -0.000000000000000000, -0.000000000000000000, 1.000000000000000000 ) ) ;
#3003=EDGE_LOOP ( 'NONE', ( #5120, #2599, #2528, #4172 ) ) ;
#3014=CARTESIAN_POINT ( 'NONE',  ( 5.000000000000000000, 5.000000000000000000, 145.0000000000000284 ) ) ;
#3017=ORIENTED_EDGE ( 'NONE', *, *, #445, .T. ) ;
#3019=VECTOR ( 'NONE', #673, 1000.000000000000000 ) ;
#3041=ORIENTED_EDGE ( 'NONE', *, *, #4660, .T. ) ;
#3042=ADVANCED_FACE ( 'NONE', ( #6998 ), #4540, .F. ) ;
#3045=LINE ( 'NONE', #2445, #4771 ) ;
#3048=ORIENTED_EDGE ( 'NONE', *, *, #363, .F. ) ;
#3049=AXIS2_PLACEMENT_3D ( 'NONE', #6700, #662, #5956 ) ;
#3056=EDGE_CURVE ( 'NONE', #6062, #3186, #7618, .T. ) ;
#3059=DIRECTION ( 'NONE',  ( -1.000000000000000000, 0.000000000000000000, 0.000000000000000000 ) ) ;
#3068=CARTESIAN_POINT ( 'NONE',  ( 259.0000000000000000, 5.000000000000001776, 140.0000000000000000 ) ) ;
#3069=FACE_OUTER_BOUND ( 'NONE', #2941, .T. ) ;
#3070=ORIENTED_EDGE ( 'NONE', *, *, #1374, .F. ) ;
#3073=CARTESIAN_POINT ( 'NONE',  ( 5.000000000000001776, -4.999999999999998224, 140.0000000000000000 ) ) ;
#3075=VERTEX_POINT ( 'NONE', #1084 ) ;
#3083=ADVANCED_FACE ( 'NONE', ( #540 ), #3649, .F. ) ;
#3091=AXIS2_PLACEMENT_3D ( 'NONE', #1335, #8140, #241 ) ;
#3094=CARTESIAN_POINT ( 'NONE',  ( 434.9999999999999432, 5.000000000000001776, 145.0000000000000284 ) ) ;
#3095=CARTESIAN_POINT ( 'NONE',  ( 53.33333333333330017, -20.00000000000000000, 162.5000000000000853 ) ) ;
#3098=DIRECTION ( 'NONE',  ( -0.000000000000000000, -0.000000000000000000, 1.000000000000000000 ) ) ;
#3105=VECTOR ( 'NONE', #5132, 1000.000000000000000 ) ;
#3107=LINE ( 'NONE', #4410, #7881 ) ;
#3123=CARTESIAN_POINT ( 'NONE',  ( 0.000000000000000000, 0.000000000000000000, 0.000000000000000000 ) ) ;
#3129=DIRECTION ( 'NONE',  ( 1.734723475976807587E-16, 1.000000000000000000, 0.000000000000000000 ) ) ;
#3130=LINE ( 'NONE', #333, #7133 ) ;
#3131=DIRECTION ( 'NONE',  ( 1.000000000000000000, 0.000000000000000000, 0.000000000000000000 ) ) ;
#3137=EDGE_LOOP ( 'NONE', ( #7036, #7537 ) ) ;
#3140=FACE_OUTER_BOUND ( 'NONE', #5030, .T. ) ;
#3144=VERTEX_POINT ( 'NONE', #1656 ) ;
#3145=VECTOR ( 'NONE', #6388, 1000.000000000000000 ) ;
#3150=VECTOR ( 'NONE', #5506, 1000.000000000000000 ) ;
#3153=CARTESIAN_POINT ( 'NONE',  ( 386.6666666666666288, -20.00000000000000000, 162.5000000000000853 ) ) ;
#3161=VECTOR ( 'NONE', #2172, 1000.000000000000000 ) ;
#3170=EDGE_CURVE ( 'NONE', #5755, #6062, #1940, .T. ) ;
#3177=VERTEX_POINT ( 'NONE', #1406 ) ;
#3180=FACE_OUTER_BOUND ( 'NONE', #5722, .T. ) ;
#3186=VERTEX_POINT ( 'NONE', #3330 ) ;
#3199=FACE_OUTER_BOUND ( 'NONE', #4594, .T. ) ;
#3209=VERTEX_POINT ( 'NONE', #1362 ) ;
#3211=DIRECTION ( 'NONE',  ( -0.000000000000000000, -0.000000000000000000, 1.000000000000000000 ) ) ;
#3214=LINE ( 'NONE', #8571, #5177 ) ;
#3218=ORIENTED_EDGE ( 'NONE', *, *, #2182, .T. ) ;
#3223=CARTESIAN_POINT ( 'NONE',  ( 181.0000000000000000, -4.999999999999998224, 145.0000000000000284 ) ) ;
#3228=EDGE_CURVE ( 'NONE', #7056, #5804, #8125, .T. ) ;
#3230=EDGE_LOOP ( 'NONE', ( #4334, #6713, #2519, #1534 ) ) ;
#3234=VECTOR ( 'NONE', #3894, 1000.000000000000000 ) ;
#3238=CIRCLE ( 'NONE', #592, 2.649999999999985700 ) ;
#3242=LINE ( 'NONE', #5881, #3396 ) ;
#3247=VERTEX_POINT ( 'NONE', #4802 ) ;
#3258=AXIS2_PLACEMENT_3D ( 'NONE', #8368, #3743, #3835 ) ;
#3264=DIRECTION ( 'NONE',  ( 0.000000000000000000, 1.000000000000000000, 0.000000000000000000 ) ) ;
#3265=PLANE ( 'NONE',  #7734 ) ;
#3266=CARTESIAN_POINT ( 'NONE',  ( 444.9999999999999432, -4.999999999999998224, 145.0000000000000284 ) ) ;
#3272=EDGE_CURVE ( 'NONE', #7609, #5626, #4300, .T. ) ;
#3288=( NAMED_UNIT ( * ) SI_UNIT ( $, .STERADIAN. ) SOLID_ANGLE_UNIT ( ) );
#3292=LINE ( 'NONE', #8520, #4355 ) ;
#3304=EDGE_LOOP ( 'NONE', ( #1436, #4905, #698, #5868, #375, #7779 ) ) ;
#3314=ORIENTED_EDGE ( 'NONE', *, *, #1263, .T. ) ;
#3316=AXIS2_PLACEMENT_3D ( 'NONE', #2880, #4103, #259 ) ;
#3322=UNCERTAINTY_MEASURE_WITH_UNIT (LENGTH_MEASURE( 1.000000000000000082E-05 ), #4689, 'distance_accuracy_value', 'NONE');
#3323=EDGE_CURVE ( 'NONE', #186, #8517, #4849, .T. ) ;
#3326=CARTESIAN_POINT ( 'NONE',  ( 219.9999999999999716, -14.99999999999999822, 165.1500000000000625 ) ) ;
#3330=CARTESIAN_POINT ( 'NONE',  ( 303.3333333333333144, -14.99999999999999822, 165.1500000000000625 ) ) ;
#3346=ORIENTED_EDGE ( 'NONE', *, *, #7790, .F. ) ;
#3348=EDGE_CURVE ( 'NONE', #2875, #4853, #2290, .T. ) ;
#3358=PLANE ( 'NONE',  #7606 ) ;
#3359=CARTESIAN_POINT ( 'NONE',  ( 269.0000000000000000, -4.999999999999998224, 140.0000000000000000 ) ) ;
#3379=EDGE_CURVE ( 'NONE', #1907, #2249, #6386, .T. ) ;
#3389=CARTESIAN_POINT ( 'NONE',  ( 386.6666666666666288, -20.00000000000000000, 162.5000000000000853 ) ) ;
#3395=DIRECTION ( 'NONE',  ( 0.000000000000000000, -1.000000000000000000, 0.000000000000000000 ) ) ;
#3396=VECTOR ( 'NONE', #2589, 1000.000000000000000 ) ;
#3400=EDGE_LOOP ( 'NONE', ( #4247, #2032 ) ) ;
#3401=FACE_OUTER_BOUND ( 'NONE', #3304, .T. ) ;
#3406=CARTESIAN_POINT ( 'NONE',  ( 347.0000000000000000, -4.999999999999998224, 140.0000000000000000 ) ) ;
#3407=DIRECTION ( 'NONE',  ( -1.734723475976807587E-16, 1.000000000000000000, 0.000000000000000000 ) ) ;
#3423=CIRCLE ( 'NONE', #503, 2.649999999999985700 ) ;
#3443=PLANE ( 'NONE',  #6983 ) ;
#3447=CARTESIAN_POINT ( 'NONE',  ( 53.33333333333330017, -15.00000000000000000, 159.8500000000001080 ) ) ;
#3452=ADVANCED_BREP_SHAPE_REPRESENTATION ( '', ( #4654, #594 ), #2832 ) ;
#3455=EDGE_CURVE ( 'NONE', #5745, #2774, #8504, .T. ) ;
#3461=VERTEX_POINT ( 'NONE', #4369 ) ;
#3462=EDGE_LOOP ( 'NONE', ( #3774, #4404, #4858, #6975 ) ) ;
#3466=CIRCLE ( 'NONE', #8197, 2.649999999999985700 ) ;
#3468=EDGE_LOOP ( 'NONE', ( #3591, #1421, #8093, #8438 ) ) ;
#3469=DIRECTION ( 'NONE',  ( -0.000000000000000000, -0.000000000000000000, 1.000000000000000000 ) ) ;
#3473=CARTESIAN_POINT ( 'NONE',  ( -4.999999999999998224, 5.000000000000001776, 140.0000000000000000 ) ) ;
#3478=ORIENTED_EDGE ( 'NONE', *, *, #4246, .F. ) ;
#3479=LINE ( 'NONE', #149, #2284 ) ;
#3482=FACE_OUTER_BOUND ( 'NONE', #3230, .T. ) ;
#3492=EDGE_CURVE ( 'NONE', #7186, #4726, #6406, .T. ) ;
#3496=FACE_BOUND ( 'NONE', #6985, .T. ) ;
#3499=DIRECTION ( 'NONE',  ( -0.000000000000000000, -0.000000000000000000, 1.000000000000000000 ) ) ;
#3505=VERTEX_POINT ( 'NONE', #5227 ) ;
#3513=FACE_OUTER_BOUND ( 'NONE', #7873, .T. ) ;
#3517=VECTOR ( 'NONE', #1880, 1000.000000000000000 ) ;
#3520=CARTESIAN_POINT ( 'NONE',  ( -30.00000000000002842, -20.00000000000000000, 140.0000000000000000 ) ) ;
#3522=AXIS2_PLACEMENT_3D ( 'NONE', #5077, #3129, #3775 ) ;
#3531=LINE ( 'NONE', #6178, #898 ) ;
#3537=DIRECTION ( 'NONE',  ( 0.000000000000000000, 0.000000000000000000, 1.000000000000000000 ) ) ;
#3540=LINE ( 'NONE', #928, #3934 ) ;
#3545=CARTESIAN_POINT ( 'NONE',  ( -30.00000000000000000, 15.00000000000000000, 140.0000000000000000 ) ) ;
#3552=AXIS2_PLACEMENT_3D ( 'NONE', #1210, #7082, #7166 ) ;
#3556=CARTESIAN_POINT ( 'NONE',  ( 470.0000000000000000, -15.00000000000000000, 180.0000000000000284 ) ) ;
#3557=ORIENTED_EDGE ( 'NONE', *, *, #3938, .F. ) ;
#3564=ADVANCED_FACE ( 'NONE', ( #3069 ), #5710, .F. ) ;
#3565=EDGE_CURVE ( 'NONE', #6024, #3923, #5268, .T. ) ;
#3571=CARTESIAN_POINT ( 'NONE',  ( 470.0000000000000000, 15.00000000000000000, 145.0000000000000284 ) ) ;
#3572=ORIENTED_EDGE ( 'NONE', *, *, #8476, .F. ) ;
#3575=AXIS2_PLACEMENT_3D ( 'NONE', #1764, #978, #6454 ) ;
#3581=CYLINDRICAL_SURFACE ( 'NONE', #4441, 2.649999999999985700 ) ;
#3589=LINE ( 'NONE', #3545, #4667 ) ;
#3591=ORIENTED_EDGE ( 'NONE', *, *, #3594, .T. ) ;
#3594=EDGE_CURVE ( 'NONE', #4134, #2451, #125, .T. ) ;
#3597=ORIENTED_EDGE ( 'NONE', *, *, #7668, .F. ) ;
#3602=VERTEX_POINT ( 'NONE', #1313 ) ;
#3606=CARTESIAN_POINT ( 'NONE',  ( 347.0000000000000000, 5.000000000000001776, 140.0000000000000000 ) ) ;
#3608=VECTOR ( 'NONE', #8470, 1000.000000000000000 ) ;
#3613=VERTEX_POINT ( 'NONE', #4617 ) ;
#3618=FACE_BOUND ( 'NONE', #8040, .T. ) ;
#3620=CARTESIAN_POINT ( 'NONE',  ( 53.33333333333330017, -15.00000000000000000, 162.5000000000000853 ) ) ;
#3623=LINE ( 'NONE', #8251, #4579 ) ;
#3648=DIRECTION ( 'NONE',  ( 0.000000000000000000, -1.000000000000000000, 0.000000000000000000 ) ) ;
#3649=CYLINDRICAL_SURFACE ( 'NONE', #406, 2.649999999999985700 ) ;
#3652=DIRECTION ( 'NONE',  ( -1.734723475976807341E-16, 1.000000000000000000, 0.000000000000000000 ) ) ;
#3662=COLOUR_RGB ( '',0.8941176470588234615, 0.8941176470588234615, 0.8941176470588234615 ) ;
#3663=CARTESIAN_POINT ( 'NONE',  ( 386.6666666666666288, -14.99999999999999822, 162.5000000000000853 ) ) ;
#3666=FACE_BOUND ( 'NONE', #4928, .T. ) ;
#3670=CIRCLE ( 'NONE', #1442, 2.649999999999985700 ) ;
#3693=LINE ( 'NONE', #6432, #5772 ) ;
#3694=DIRECTION ( 'NONE',  ( -0.000000000000000000, 1.000000000000000000, -0.000000000000000000 ) ) ;
#3700=VERTEX_POINT ( 'NONE', #7227 ) ;
#3702=CARTESIAN_POINT ( 'NONE',  ( 93.00000000000000000, -4.999999999999998224, 145.0000000000000284 ) ) ;
#3709=CARTESIAN_POINT ( 'NONE',  ( 170.9999999999999716, -4.999999999999998224, 139.9990000000000236 ) ) ;
#3713=VECTOR ( 'NONE', #7188, 1000.000000000000000 ) ;
#3715=LINE ( 'NONE', #5059, #1821 ) ;
#3718=ORIENTED_EDGE ( 'NONE', *, *, #1149, .T. ) ;
#3720=ADVANCED_FACE ( 'NONE', ( #6134, #2971, #6839, #2191, #3666, #6227, #8119 ), #970, .T. ) ;
#3743=DIRECTION ( 'NONE',  ( 1.000000000000000000, 1.734723475976807587E-16, 0.000000000000000000 ) ) ;
#3752=FACE_OUTER_BOUND ( 'NONE', #8259, .T. ) ;
#3754=ADVANCED_FACE ( 'NONE', ( #4969 ), #3581, .F. ) ;
#3760=ORIENTED_EDGE ( 'NONE', *, *, #1575, .F. ) ;
#3764=DIRECTION ( 'NONE',  ( -1.734723475976807587E-16, 1.000000000000000000, 0.000000000000000000 ) ) ;
#3766=ADVANCED_FACE ( 'NONE', ( #6270, #5571, #5442, #3496, #7538, #2925 ), #4274, .F. ) ;
#3773=ORIENTED_EDGE ( 'NONE', *, *, #706, .F. ) ;
#3774=ORIENTED_EDGE ( 'NONE', *, *, #2663, .T. ) ;
#3775=DIRECTION ( 'NONE',  ( -1.000000000000000000, 1.734723475976807587E-16, 0.000000000000000000 ) ) ;
#3785=ORIENTED_EDGE ( 'NONE', *, *, #363, .T. ) ;
#3788=CARTESIAN_POINT ( 'NONE',  ( 219.9999999999999716, -15.00000000000000000, 165.1500000000000625 ) ) ;
#3793=ORIENTED_EDGE ( 'NONE', *, *, #2375, .T. ) ;
#3800=VECTOR ( 'NONE', #6337, 1000.000000000000000 ) ;
#3801=VECTOR ( 'NONE', #1212, 1000.000000000000000 ) ;
#3803=CARTESIAN_POINT ( 'NONE',  ( 434.9999999999999432, 5.000000000000001776, 145.0000000000000284 ) ) ;
#3805=EDGE_CURVE ( 'NONE', #5804, #3177, #1581, .T. ) ;
#3808=EDGE_CURVE ( 'NONE', #1549, #7220, #2283, .T. ) ;
#3821=VECTOR ( 'NONE', #4167, 1000.000000000000000 ) ;
#3829=LINE ( 'NONE', #6476, #156 ) ;
#3833=DIRECTION ( 'NONE',  ( 1.000000000000000000, 1.734723475976807587E-16, 0.000000000000000000 ) ) ;
#3834=ADVANCED_FACE ( 'NONE', ( #2369 ), #8332, .F. ) ;
#3835=DIRECTION ( 'NONE',  ( -1.734723475976807587E-16, 1.000000000000000000, 0.000000000000000000 ) ) ;
#3849=DIRECTION ( 'NONE',  ( 0.000000000000000000, 0.000000000000000000, 1.000000000000000000 ) ) ;
#3859=ORIENTED_EDGE ( 'NONE', *, *, #849, .F. ) ;
#3866=CARTESIAN_POINT ( 'NONE',  ( 434.9999999999999432, -4.999999999999998224, 140.0000000000000000 ) ) ;
#3869=PLANE ( 'NONE',  #3552 ) ;
#3892=CARTESIAN_POINT ( 'NONE',  ( 259.0000000000000000, 5.000000000000001776, 145.0000000000000284 ) ) ;
#3894=DIRECTION ( 'NONE',  ( -1.734723475976807587E-16, 1.000000000000000000, 0.000000000000000000 ) ) ;
#3901=ORIENTED_EDGE ( 'NONE', *, *, #6636, .T. ) ;
#3923=VERTEX_POINT ( 'NONE', #7414 ) ;
#3934=VECTOR ( 'NONE', #174, 1000.000000000000000 ) ;
#3938=EDGE_CURVE ( 'NONE', #3209, #7011, #7942, .T. ) ;
#3947=ORIENTED_EDGE ( 'NONE', *, *, #67, .T. ) ;
#3950=ORIENTED_EDGE ( 'NONE', *, *, #7126, .T. ) ;
#3959=CIRCLE ( 'NONE', #8416, 2.649999999999985700 ) ;
#3968=CARTESIAN_POINT ( 'NONE',  ( 170.9999999999999716, -4.999999999999998224, 139.9990000000000236 ) ) ;
#3974=CARTESIAN_POINT ( 'NONE',  ( 347.0000000000000000, 5.000000000000001776, 140.0000000000000000 ) ) ;
#3977=DIRECTION ( 'NONE',  ( -1.734723475976807587E-16, 1.000000000000000000, 0.000000000000000000 ) ) ;
#3978=LINE ( 'NONE', #667, #1427 ) ;
#3982=LINE ( 'NONE', #7158, #1281 ) ;
#3985=CARTESIAN_POINT ( 'NONE',  ( 269.0000000000000000, 5.000000000000000000, 139.9990000000000236 ) ) ;
#3988=ORIENTED_EDGE ( 'NONE', *, *, #4865, .F. ) ;
#3995=AXIS2_PLACEMENT_3D ( 'NONE', #495, #4494, #1894 ) ;
#4000=PLANE ( 'NONE',  #1203 ) ;
#4002=FACE_BOUND ( 'NONE', #722, .T. ) ;
#4003=ORIENTED_EDGE ( 'NONE', *, *, #7571, .T. ) ;
#4004=EDGE_LOOP ( 'NONE', ( #4516, #3950, #1386, #4946 ) ) ;
#4006=DIRECTION ( 'NONE',  ( -1.734723475976807587E-16, 1.000000000000000000, 0.000000000000000000 ) ) ;
#4012=AXIS2_PLACEMENT_3D ( 'NONE', #7844, #8018, #2011 ) ;
#4015=LINE ( 'NONE', #3359, #1223 ) ;
#4028=VERTEX_POINT ( 'NONE', #2930 ) ;
#4037=EDGE_LOOP ( 'NONE', ( #2293, #2094, #5778, #3314 ) ) ;
#4045=CARTESIAN_POINT ( 'NONE',  ( 181.0000000000000000, -4.999999999999998224, 139.9990000000000236 ) ) ;
#4046=DIRECTION ( 'NONE',  ( -1.000000000000000000, 1.734723475976807587E-16, 0.000000000000000000 ) ) ;
#4052=DIRECTION ( 'NONE',  ( -0.000000000000000000, 1.000000000000000000, -0.000000000000000000 ) ) ;
#4053=CARTESIAN_POINT ( 'NONE',  ( 93.00000000000000000, 5.000000000000000000, 140.0000000000000000 ) ) ;
#4056=ORIENTED_EDGE ( 'NONE', *, *, #4975, .F. ) ;
#4059=EDGE_CURVE ( 'NONE', #5369, #8255, #2978, .T. ) ;
#4070=ORIENTED_EDGE ( 'NONE', *, *, #8432, .T. ) ;
#4085=( NAMED_UNIT ( * ) SI_UNIT ( $, .STERADIAN. ) SOLID_ANGLE_UNIT ( ) );
#4086=ORIENTED_EDGE ( 'NONE', *, *, #4538, .F. ) ;
#4098=ORIENTED_EDGE ( 'NONE', *, *, #2229, .T. ) ;
#4103=DIRECTION ( 'NONE',  ( -1.000000000000000000, 0.000000000000000000, 0.000000000000000000 ) ) ;
#4108=DIRECTION ( 'NONE',  ( -0.000000000000000000, 1.000000000000000000, -0.000000000000000000 ) ) ;
#4109=DIRECTION ( 'NONE',  ( -1.734723475976807341E-16, 1.000000000000000000, 0.000000000000000000 ) ) ;
#4126=VECTOR ( 'NONE', #4109, 1000.000000000000000 ) ;
#4128=VECTOR ( 'NONE', #4747, 1000.000000000000000 ) ;
#4134=VERTEX_POINT ( 'NONE', #2238 ) ;
#4151=ORIENTED_EDGE ( 'NONE', *, *, #202, .F. ) ;
#4152=EDGE_LOOP ( 'NONE', ( #5280, #1640, #7829, #5540 ) ) ;
#4163=CARTESIAN_POINT ( 'NONE',  ( 470.0000000000000000, -20.00000000000000000, 180.0000000000000284 ) ) ;
#4164=VERTEX_POINT ( 'NONE', #7595 ) ;
#4167=DIRECTION ( 'NONE',  ( -1.000000000000000000, 1.734723475976807587E-16, 0.000000000000000000 ) ) ;
#4172=ORIENTED_EDGE ( 'NONE', *, *, #2311, .F. ) ;
#4173=EDGE_CURVE ( 'NONE', #2638, #5335, #3623, .T. ) ;
#4191=VERTEX_POINT ( 'NONE', #3068 ) ;
#4192=ORIENTED_EDGE ( 'NONE', *, *, #6939, .T. ) ;
#4193=EDGE_CURVE ( 'NONE', #6781, #5745, #5752, .T. ) ;
#4216=AXIS2_PLACEMENT_3D ( 'NONE', #1294, #4474, #7131 ) ;
#4217=CARTESIAN_POINT ( 'NONE',  ( 347.0000000000000000, -4.999999999999998224, 140.0000000000000000 ) ) ;
#4218=CARTESIAN_POINT ( 'NONE',  ( 181.0000000000000000, -4.999999999999998224, 140.0000000000000000 ) ) ;
#4230=ORIENTED_EDGE ( 'NONE', *, *, #1244, .T. ) ;
#4234=DIRECTION ( 'NONE',  ( 0.000000000000000000, 1.000000000000000000, 0.000000000000000000 ) ) ;
#4239=DIRECTION ( 'NONE',  ( -1.734723475976807341E-16, 1.000000000000000000, 0.000000000000000000 ) ) ;
#4241=ORIENTED_EDGE ( 'NONE', *, *, #706, .T. ) ;
#4246=EDGE_CURVE ( 'NONE', #2638, #3461, #7060, .T. ) ;
#4247=ORIENTED_EDGE ( 'NONE', *, *, #6939, .F. ) ;
#4249=VERTEX_POINT ( 'NONE', #1145 ) ;
#4250=( NAMED_UNIT ( * ) PLANE_ANGLE_UNIT ( ) SI_UNIT ( $, .RADIAN. ) );
#4252=PRODUCT_CONTEXT ( 'NONE', #6415, 'mechanical' ) ;
#4255=LINE ( 'NONE', #2866, #6141 ) ;
#4256=CYLINDRICAL_SURFACE ( 'NONE', #6153, 2.649999999999985700 ) ;
#4271=CARTESIAN_POINT ( 'NONE',  ( 434.9999999999999432, 5.000000000000001776, 140.0000000000000000 ) ) ;
#4274=PLANE ( 'NONE',  #1808 ) ;
#4286=ORIENTED_EDGE ( 'NONE', *, *, #5570, .T. ) ;
#4288=LINE ( 'NONE', #5110, #749 ) ;
#4294=DIRECTION ( 'NONE',  ( 0.000000000000000000, -1.000000000000000000, 0.000000000000000000 ) ) ;
#4297=EDGE_LOOP ( 'NONE', ( #7599, #4151, #3947, #1204 ) ) ;
#4300=CIRCLE ( 'NONE', #539, 2.649999999999985700 ) ;
#4307=DIRECTION ( 'NONE',  ( -1.734723475976807587E-16, 1.000000000000000000, 0.000000000000000000 ) ) ;
#4312=CARTESIAN_POINT ( 'NONE',  ( 93.00000000000000000, -4.999999999999998224, 139.9990000000000236 ) ) ;
#4314=LINE ( 'NONE', #1531, #1911 ) ;
#4317=DIRECTION ( 'NONE',  ( 0.000000000000000000, 1.000000000000000000, 0.000000000000000000 ) ) ;
#4326=ORIENTED_EDGE ( 'NONE', *, *, #445, .F. ) ;
#4330=EDGE_CURVE ( 'NONE', #2249, #3505, #3715, .T. ) ;
#4334=ORIENTED_EDGE ( 'NONE', *, *, #2002, .F. ) ;
#4340=DIRECTION ( 'NONE',  ( 0.000000000000000000, 0.000000000000000000, 1.000000000000000000 ) ) ;
#4346=AXIS2_PLACEMENT_3D ( 'NONE', #5532, #6794, #8205 ) ;
#4349=EDGE_LOOP ( 'NONE', ( #1725, #6374 ) ) ;
#4355=VECTOR ( 'NONE', #2601, 1000.000000000000000 ) ;
#4358=CARTESIAN_POINT ( 'NONE',  ( 170.9999999999999716, 5.000000000000001776, 140.0000000000000000 ) ) ;
#4360=EDGE_CURVE ( 'NONE', #5286, #6478, #7792, .T. ) ;
#4361=DIRECTION ( 'NONE',  ( 0.000000000000000000, 0.000000000000000000, 1.000000000000000000 ) ) ;
#4365=CARTESIAN_POINT ( 'NONE',  ( -4.999999999999998224, -4.999999999999998224, 139.9990000000000236 ) ) ;
#4369=CARTESIAN_POINT ( 'NONE',  ( 170.9999999999999716, -4.999999999999998224, 140.0000000000000000 ) ) ;
#4370=CARTESIAN_POINT ( 'NONE',  ( 259.0000000000000000, -4.999999999999998224, 139.9990000000000236 ) ) ;
#4376=DIRECTION ( 'NONE',  ( -0.000000000000000000, -0.000000000000000000, 1.000000000000000000 ) ) ;
#4381=ORIENTED_EDGE ( 'NONE', *, *, #7415, .F. ) ;
#4382=FILL_AREA_STYLE_COLOUR ( '', #3662 ) ;
#4396=EDGE_CURVE ( 'NONE', #4853, #5335, #2958, .T. ) ;
#4404=ORIENTED_EDGE ( 'NONE', *, *, #4360, .T. ) ;
#4410=CARTESIAN_POINT ( 'NONE',  ( 259.0000000000000000, 5.000000000000001776, 145.0000000000000284 ) ) ;
#4420=EDGE_LOOP ( 'NONE', ( #2853, #8009, #4877, #3773 ) ) ;
#4441=AXIS2_PLACEMENT_3D ( 'NONE', #3620, #2148, #3537 ) ;
#4459=ADVANCED_FACE ( 'NONE', ( #7002 ), #6260, .F. ) ;
#4460=ORIENTED_EDGE ( 'NONE', *, *, #6210, .F. ) ;
#4474=DIRECTION ( 'NONE',  ( 0.000000000000000000, 0.000000000000000000, -1.000000000000000000 ) ) ;
#4476=ORIENTED_EDGE ( 'NONE', *, *, #5828, .F. ) ;
#4477=PLANE ( 'NONE',  #7703 ) ;
#4490=VECTOR ( 'NONE', #547, 1000.000000000000000 ) ;
#4494=DIRECTION ( 'NONE',  ( -0.000000000000000000, 1.000000000000000000, -0.000000000000000000 ) ) ;
#4506=ORIENTED_EDGE ( 'NONE', *, *, #6988, .F. ) ;
#4516=ORIENTED_EDGE ( 'NONE', *, *, #4059, .T. ) ;
#4517=CARTESIAN_POINT ( 'NONE',  ( 82.99999999999998579, -4.999999999999998224, 140.0000000000000000 ) ) ;
#4520=DIRECTION ( 'NONE',  ( -1.734723475976807587E-16, 1.000000000000000000, 0.000000000000000000 ) ) ;
#4536=ADVANCED_FACE ( 'NONE', ( #2609, #601, #5290, #8574, #4554, #4002, #5210 ), #5983, .F. ) ;
#4538=EDGE_CURVE ( 'NONE', #2983, #2875, #3829, .T. ) ;
#4540=CYLINDRICAL_SURFACE ( 'NONE', #111, 2.649999999999985700 ) ;
#4549=CARTESIAN_POINT ( 'NONE',  ( -30.00000000000002842, -20.00000000000000000, 180.0000000000000284 ) ) ;
#4554=FACE_BOUND ( 'NONE', #4989, .T. ) ;
#4558=CARTESIAN_POINT ( 'NONE',  ( 347.0000000000000000, -4.999999999999998224, 139.9990000000000236 ) ) ;
#4562=ORIENTED_EDGE ( 'NONE', *, *, #2177, .F. ) ;
#4566=EDGE_LOOP ( 'NONE', ( #5291, #254, #5810, #7965 ) ) ;
#4579=VECTOR ( 'NONE', #3499, 1000.000000000000000 ) ;
#4583=CARTESIAN_POINT ( 'NONE',  ( 434.9999999999999432, -4.999999999999998224, 140.0000000000000000 ) ) ;
#4591=ADVANCED_FACE ( 'NONE', ( #2650 ), #7962, .F. ) ;
#4594=EDGE_LOOP ( 'NONE', ( #7105, #7687, #7387, #1185 ) ) ;
#4597=ORIENTED_EDGE ( 'NONE', *, *, #1456, .F. ) ;
#4603=VECTOR ( 'NONE', #3977, 1000.000000000000000 ) ;
#4614=CARTESIAN_POINT ( 'NONE',  ( -30.00000000000000000, -15.00000000000000000, 145.0000000000000284 ) ) ;
#4615=FACE_OUTER_BOUND ( 'NONE', #4297, .T. ) ;
#4617=CARTESIAN_POINT ( 'NONE',  ( 93.00000000000000000, 5.000000000000000000, 145.0000000000000284 ) ) ;
#4626=EDGE_CURVE ( 'NONE', #4892, #6564, #5423, .T. ) ;
#4632=ORIENTED_EDGE ( 'NONE', *, *, #2503, .T. ) ;
#4640=AXIS2_PLACEMENT_3D ( 'NONE', #4558, #2087, #692 ) ;
#4653=EDGE_LOOP ( 'NONE', ( #5843, #448, #8194, #7167 ) ) ;
#4654=MANIFOLD_SOLID_BREP ( 'M5 Clearance Hole1', #8448 ) ;
#4656=FACE_OUTER_BOUND ( 'NONE', #5777, .T. ) ;
#4660=EDGE_CURVE ( 'NONE', #7555, #7704, #7431, .T. ) ;
#4661=LINE ( 'NONE', #1937, #7826 ) ;
#4665=CARTESIAN_POINT ( 'NONE',  ( 259.0000000000000000, -4.999999999999998224, 145.0000000000000284 ) ) ;
#4667=VECTOR ( 'NONE', #5452, 1000.000000000000000 ) ;
#4669=DIRECTION ( 'NONE',  ( -0.000000000000000000, -1.000000000000000000, -0.000000000000000000 ) ) ;
#4670=VECTOR ( 'NONE', #4052, 1000.000000000000000 ) ;
#4675=UNCERTAINTY_MEASURE_WITH_UNIT (LENGTH_MEASURE( 1.000000000000000082E-05 ), #6248, 'distance_accuracy_value', 'NONE');
#4676=ORIENTED_EDGE ( 'NONE', *, *, #7528, .T. ) ;
#4685=LINE ( 'NONE', #5898, #3801 ) ;
#4689=( LENGTH_UNIT ( ) NAMED_UNIT ( * ) SI_UNIT ( .MILLI., .METRE. ) );
#4692=DIRECTION ( 'NONE',  ( 1.000000000000000000, 0.000000000000000000, 0.000000000000000000 ) ) ;
#4695=CARTESIAN_POINT ( 'NONE',  ( 82.99999999999998579, 5.000000000000001776, 139.9990000000000236 ) ) ;
#4726=VERTEX_POINT ( 'NONE', #575 ) ;
#4730=ADVANCED_FACE ( 'NONE', ( #3199 ), #5833, .F. ) ;
#4735=VERTEX_POINT ( 'NONE', #3892 ) ;
#4739=CARTESIAN_POINT ( 'NONE',  ( 170.9999999999999716, -4.999999999999998224, 140.0000000000000000 ) ) ;
#4745=ORIENTED_EDGE ( 'NONE', *, *, #3379, .T. ) ;
#4747=DIRECTION ( 'NONE',  ( 0.000000000000000000, 1.000000000000000000, 0.000000000000000000 ) ) ;
#4748=LINE ( 'NONE', #6532, #2486 ) ;
#4749=ORIENTED_EDGE ( 'NONE', *, *, #7064, .F. ) ;
#4753=( GEOMETRIC_REPRESENTATION_CONTEXT ( 3 ) GLOBAL_UNCERTAINTY_ASSIGNED_CONTEXT ( ( #3322 ) ) GLOBAL_UNIT_ASSIGNED_CONTEXT ( ( #4689, #6773, #4085 ) ) REPRESENTATION_CONTEXT ( 'NONE', 'WORKASPACE' ) );
#4759=EDGE_CURVE ( 'NONE', #951, #4853, #7278, .T. ) ;
#4768=DIRECTION ( 'NONE',  ( -0.000000000000000000, 1.000000000000000000, -0.000000000000000000 ) ) ;
#4771=VECTOR ( 'NONE', #1125, 1000.000000000000000 ) ;
#4782=DIRECTION ( 'NONE',  ( 0.000000000000000000, 0.000000000000000000, 1.000000000000000000 ) ) ;
#4785=DIRECTION ( 'NONE',  ( -0.000000000000000000, -0.000000000000000000, 1.000000000000000000 ) ) ;
#4787=ORIENTED_EDGE ( 'NONE', *, *, #7720, .F. ) ;
#4790=ORIENTED_EDGE ( 'NONE', *, *, #5724, .T. ) ;
#4795=FACE_BOUND ( 'NONE', #3400, .T. ) ;
#4797=DIRECTION ( 'NONE',  ( -1.000000000000000000, 0.000000000000000000, 0.000000000000000000 ) ) ;
#4802=CARTESIAN_POINT ( 'NONE',  ( 219.9999999999999716, -20.00000000000000000, 159.8500000000001080 ) ) ;
#4807=EDGE_CURVE ( 'NONE', #7011, #5482, #4661, .T. ) ;
#4814=ORIENTED_EDGE ( 'NONE', *, *, #4330, .F. ) ;
#4815=DIRECTION ( 'NONE',  ( 0.000000000000000000, -1.000000000000000000, 0.000000000000000000 ) ) ;
#4816=ORIENTED_EDGE ( 'NONE', *, *, #2946, .F. ) ;
#4827=DIRECTION ( 'NONE',  ( 0.000000000000000000, -0.000000000000000000, 1.000000000000000000 ) ) ;
#4831=EDGE_LOOP ( 'NONE', ( #1078, #124, #7077, #2439, #4241, #429 ) ) ;
#4840=FACE_BOUND ( 'NONE', #7994, .T. ) ;
#4849=LINE ( 'NONE', #6189, #2371 ) ;
#4853=VERTEX_POINT ( 'NONE', #1316 ) ;
#4855=AXIS2_PLACEMENT_3D ( 'NONE', #1492, #1622, #170 ) ;
#4858=ORIENTED_EDGE ( 'NONE', *, *, #6565, .F. ) ;
#4865=EDGE_CURVE ( 'NONE', #186, #819, #3978, .T. ) ;
#4875=CARTESIAN_POINT ( 'NONE',  ( 357.0000000000000000, 5.000000000000000000, 140.0000000000000000 ) ) ;
#4877=ORIENTED_EDGE ( 'NONE', *, *, #3228, .F. ) ;
#4887=CARTESIAN_POINT ( 'NONE',  ( 82.99999999999998579, -4.999999999999998224, 140.0000000000000000 ) ) ;
#4892=VERTEX_POINT ( 'NONE', #1625 ) ;
#4894=ORIENTED_EDGE ( 'NONE', *, *, #7443, .F. ) ;
#4895=DIRECTION ( 'NONE',  ( -0.000000000000000000, 1.000000000000000000, -0.000000000000000000 ) ) ;
#4897=EDGE_CURVE ( 'NONE', #3177, #4028, #3540, .T. ) ;
#4901=ORIENTED_EDGE ( 'NONE', *, *, #4330, .T. ) ;
#4903=FACE_OUTER_BOUND ( 'NONE', #2158, .T. ) ;
#4905=ORIENTED_EDGE ( 'NONE', *, *, #3805, .F. ) ;
#4910=CARTESIAN_POINT ( 'NONE',  ( 82.99999999999998579, 5.000000000000001776, 140.0000000000000000 ) ) ;
#4914=ORIENTED_EDGE ( 'NONE', *, *, #551, .F. ) ;
#4916=STYLED_ITEM ( 'NONE', ( #1778 ), #3452 ) ;
#4919=ORIENTED_EDGE ( 'NONE', *, *, #3056, .F. ) ;
#4928=EDGE_LOOP ( 'NONE', ( #3793, #8526, #4070, #2481 ) ) ;
#4929=CARTESIAN_POINT ( 'NONE',  ( 82.99999999999998579, 5.000000000000001776, 139.9990000000000236 ) ) ;
#4934=CARTESIAN_POINT ( 'NONE',  ( 181.0000000000000000, 5.000000000000000000, 139.9990000000000236 ) ) ;
#4937=ORIENTED_EDGE ( 'NONE', *, *, #1949, .F. ) ;
#4944=AXIS2_PLACEMENT_3D ( 'NONE', #6445, #1883, #4520 ) ;
#4946=ORIENTED_EDGE ( 'NONE', *, *, #2311, .T. ) ;
#4948=CARTESIAN_POINT ( 'NONE',  ( 269.0000000000000000, -4.999999999999998224, 140.0000000000000000 ) ) ;
#4961=DIRECTION ( 'NONE',  ( 1.000000000000000000, 1.734723475976807587E-16, 0.000000000000000000 ) ) ;
#4969=FACE_OUTER_BOUND ( 'NONE', #2073, .T. ) ;
#4975=EDGE_CURVE ( 'NONE', #3144, #874, #5864, .T. ) ;
#4989=EDGE_LOOP ( 'NONE', ( #2368, #6082, #3346, #4914 ) ) ;
#4993=ADVANCED_FACE ( 'NONE', ( #8159 ), #6136, .T. ) ;
#4996=VECTOR ( 'NONE', #446, 1000.000000000000000 ) ;
#4997=CARTESIAN_POINT ( 'NONE',  ( 303.3333333333333144, -15.00000000000000000, 165.1500000000000625 ) ) ;
#4998=ORIENTED_EDGE ( 'NONE', *, *, #5397, .T. ) ;
#5019=ORIENTED_EDGE ( 'NONE', *, *, #2177, .T. ) ;
#5021=DIRECTION ( 'NONE',  ( 0.000000000000000000, -1.000000000000000000, 0.000000000000000000 ) ) ;
#5024=EDGE_CURVE ( 'NONE', #3247, #7213, #3238, .T. ) ;
#5027=ORIENTED_EDGE ( 'NONE', *, *, #841, .F. ) ;
#5030=EDGE_LOOP ( 'NONE', ( #3901, #208, #117, #1127 ) ) ;
#5032=DIRECTION ( 'NONE',  ( 0.000000000000000000, 0.000000000000000000, -1.000000000000000000 ) ) ;
#5034=DIRECTION ( 'NONE',  ( -1.000000000000000000, 1.734723475976807587E-16, 0.000000000000000000 ) ) ;
#5044=ORIENTED_EDGE ( 'NONE', *, *, #2865, .F. ) ;
#5045=VERTEX_POINT ( 'NONE', #5572 ) ;
#5047=CARTESIAN_POINT ( 'NONE',  ( 53.33333333333330017, -14.99999999999999822, 162.5000000000000853 ) ) ;
#5059=CARTESIAN_POINT ( 'NONE',  ( 136.6666666666666288, -15.00000000000000000, 165.1500000000000625 ) ) ;
#5060=DIRECTION ( 'NONE',  ( 0.000000000000000000, 0.000000000000000000, 1.000000000000000000 ) ) ;
#5062=EDGE_LOOP ( 'NONE', ( #7710, #4562, #4901, #386 ) ) ;
#5067=ORIENTED_EDGE ( 'NONE', *, *, #1654, .F. ) ;
#5073=ADVANCED_FACE ( 'NONE', ( #3752 ), #8501, .F. ) ;
#5077=CARTESIAN_POINT ( 'NONE',  ( 347.0000000000000000, 5.000000000000001776, 139.9990000000000236 ) ) ;
#5078=EDGE_CURVE ( 'NONE', #4892, #3700, #8464, .T. ) ;
#5080=VECTOR ( 'NONE', #3648, 1000.000000000000000 ) ;
#5086=ORIENTED_EDGE ( 'NONE', *, *, #4807, .T. ) ;
#5091=CARTESIAN_POINT ( 'NONE',  ( 136.6666666666666288, -15.00000000000000000, 162.5000000000000853 ) ) ;
#5092=AXIS2_PLACEMENT_3D ( 'NONE', #2902, #8311, #6987 ) ;
#5096=DIRECTION ( 'NONE',  ( -1.000000000000000000, 0.000000000000000000, 0.000000000000000000 ) ) ;
#5110=CARTESIAN_POINT ( 'NONE',  ( 470.0000000000000000, 15.00000000000000000, 145.0000000000000284 ) ) ;
#5115=LINE ( 'NONE', #6463, #7316 ) ;
#5120=ORIENTED_EDGE ( 'NONE', *, *, #7799, .T. ) ;
#5132=DIRECTION ( 'NONE',  ( -0.000000000000000000, 1.000000000000000000, -0.000000000000000000 ) ) ;
#5149=EDGE_CURVE ( 'NONE', #7186, #2677, #5826, .T. ) ;
#5157=ORIENTED_EDGE ( 'NONE', *, *, #681, .T. ) ;
#5168=ORIENTED_EDGE ( 'NONE', *, *, #4173, .T. ) ;
#5173=DIRECTION ( 'NONE',  ( 0.000000000000000000, 0.000000000000000000, 1.000000000000000000 ) ) ;
#5177=VECTOR ( 'NONE', #7870, 1000.000000000000000 ) ;
#5210=FACE_BOUND ( 'NONE', #2840, .T. ) ;
#5227=CARTESIAN_POINT ( 'NONE',  ( 136.6666666666666288, -14.99999999999999822, 165.1500000000000625 ) ) ;
#5232=CARTESIAN_POINT ( 'NONE',  ( 470.0000000000000000, -15.00000000000000000, 145.0000000000000284 ) ) ;
#5244=CARTESIAN_POINT ( 'NONE',  ( 82.99999999999998579, 5.000000000000001776, 140.0000000000000000 ) ) ;
#5245=ORIENTED_EDGE ( 'NONE', *, *, #2946, .T. ) ;
#5252=AXIS2_PLACEMENT_3D ( 'NONE', #3968, #610, #1257 ) ;
#5260=DIRECTION ( 'NONE',  ( 0.000000000000000000, 1.000000000000000000, 0.000000000000000000 ) ) ;
#5265=VERTEX_POINT ( 'NONE', #2619 ) ;
#5268=CIRCLE ( 'NONE', #2777, 2.649999999999985700 ) ;
#5280=ORIENTED_EDGE ( 'NONE', *, *, #1456, .T. ) ;
#5286=VERTEX_POINT ( 'NONE', #5304 ) ;
#5288=DIRECTION ( 'NONE',  ( -1.000000000000000000, 1.734723475976807587E-16, 0.000000000000000000 ) ) ;
#5290=FACE_OUTER_BOUND ( 'NONE', #4420, .T. ) ;
#5291=ORIENTED_EDGE ( 'NONE', *, *, #6565, .T. ) ;
#5304=CARTESIAN_POINT ( 'NONE',  ( 357.0000000000000000, -4.999999999999998224, 145.0000000000000284 ) ) ;
#5309=ORIENTED_EDGE ( 'NONE', *, *, #3808, .T. ) ;
#5313=CARTESIAN_POINT ( 'NONE',  ( 181.0000000000000000, -4.999999999999998224, 145.0000000000000284 ) ) ;
#5330=VECTOR ( 'NONE', #6150, 1000.000000000000000 ) ;
#5335=VERTEX_POINT ( 'NONE', #1441 ) ;
#5337=CARTESIAN_POINT ( 'NONE',  ( 444.9999999999999432, 5.000000000000000000, 140.0000000000000000 ) ) ;
#5345=CARTESIAN_POINT ( 'NONE',  ( 53.33333333333330017, -20.00000000000000000, 162.5000000000000853 ) ) ;
#5347=DIRECTION ( 'NONE',  ( 1.000000000000000000, 0.000000000000000000, 0.000000000000000000 ) ) ;
#5365=VECTOR ( 'NONE', #4239, 1000.000000000000000 ) ;
#5369=VERTEX_POINT ( 'NONE', #1571 ) ;
#5370=ORIENTED_EDGE ( 'NONE', *, *, #2865, .T. ) ;
#5374=CARTESIAN_POINT ( 'NONE',  ( 259.0000000000000000, 5.000000000000001776, 139.9990000000000236 ) ) ;
#5375=VECTOR ( 'NONE', #2869, 1000.000000000000000 ) ;
#5387=CARTESIAN_POINT ( 'NONE',  ( 82.99999999999998579, -4.999999999999998224, 145.0000000000000284 ) ) ;
#5389=LINE ( 'NONE', #4739, #517 ) ;
#5395=ADVANCED_FACE ( 'NONE', ( #877 ), #6177, .F. ) ;
#5397=EDGE_CURVE ( 'NONE', #5626, #7609, #8393, .T. ) ;
#5399=DIRECTION ( 'NONE',  ( 1.000000000000000000, 0.000000000000000000, 0.000000000000000000 ) ) ;
#5406=CARTESIAN_POINT ( 'NONE',  ( 82.99999999999998579, -4.999999999999998224, 139.9990000000000236 ) ) ;
#5416=ORIENTED_EDGE ( 'NONE', *, *, #3323, .T. ) ;
#5420=CARTESIAN_POINT ( 'NONE',  ( 434.9999999999999432, 5.000000000000001776, 139.9990000000000236 ) ) ;
#5421=SHAPE_DEFINITION_REPRESENTATION ( #6135, #7993 ) ;
#5423=LINE ( 'NONE', #6111, #6974 ) ;
#5430=ORIENTED_EDGE ( 'NONE', *, *, #7571, .F. ) ;
#5442=FACE_BOUND ( 'NONE', #7655, .T. ) ;
#5450=VECTOR ( 'NONE', #2372, 1000.000000000000000 ) ;
#5452=DIRECTION ( 'NONE',  ( 1.000000000000000000, 0.000000000000000000, 0.000000000000000000 ) ) ;
#5464=CARTESIAN_POINT ( 'NONE',  ( 259.0000000000000000, 5.000000000000001776, 140.0000000000000000 ) ) ;
#5475=CIRCLE ( 'NONE', #46, 2.649999999999985700 ) ;
#5477=DIRECTION ( 'NONE',  ( 0.000000000000000000, 0.000000000000000000, 1.000000000000000000 ) ) ;
#5478=ORIENTED_EDGE ( 'NONE', *, *, #2229, .F. ) ;
#5482=VERTEX_POINT ( 'NONE', #3702 ) ;
#5486=DIRECTION ( 'NONE',  ( 0.000000000000000000, 0.000000000000000000, 1.000000000000000000 ) ) ;
#5502=LINE ( 'NONE', #1413, #5330 ) ;
#5504=VECTOR ( 'NONE', #905, 1000.000000000000000 ) ;
#5506=DIRECTION ( 'NONE',  ( -0.000000000000000000, 1.000000000000000000, -0.000000000000000000 ) ) ;
#5522=EDGE_CURVE ( 'NONE', #7213, #6477, #5737, .T. ) ;
#5532=CARTESIAN_POINT ( 'NONE',  ( 386.6666666666666288, -14.99999999999999822, 162.5000000000000853 ) ) ;
#5533=ADVANCED_FACE ( 'NONE', ( #8414 ), #4477, .F. ) ;
#5534=AXIS2_PLACEMENT_3D ( 'NONE', #1710, #6399, #3059 ) ;
#5537=DIRECTION ( 'NONE',  ( 0.000000000000000000, 0.000000000000000000, 1.000000000000000000 ) ) ;
#5540=ORIENTED_EDGE ( 'NONE', *, *, #3492, .F. ) ;
#5564=DIRECTION ( 'NONE',  ( 0.000000000000000000, -0.000000000000000000, -1.000000000000000000 ) ) ;
#5568=PLANE ( 'NONE',  #5534 ) ;
#5570=EDGE_CURVE ( 'NONE', #8118, #2774, #8325, .T. ) ;
#5571=FACE_BOUND ( 'NONE', #2765, .T. ) ;
#5572=CARTESIAN_POINT ( 'NONE',  ( 347.0000000000000000, -4.999999999999998224, 145.0000000000000284 ) ) ;
#5576=DIRECTION ( 'NONE',  ( 0.000000000000000000, 1.000000000000000000, 0.000000000000000000 ) ) ;
#5597=ORIENTED_EDGE ( 'NONE', *, *, #1244, .F. ) ;
#5603=LINE ( 'NONE', #6821, #6186 ) ;
#5606=EDGE_CURVE ( 'NONE', #1549, #3209, #6686, .T. ) ;
#5607=VECTOR ( 'NONE', #4376, 1000.000000000000000 ) ;
#5614=AXIS2_PLACEMENT_3D ( 'NONE', #6458, #7157, #5834 ) ;
#5625=LINE ( 'NONE', #4370, #6619 ) ;
#5626=VERTEX_POINT ( 'NONE', #5987 ) ;
#5636=EDGE_LOOP ( 'NONE', ( #6220, #4816, #8183, #4192 ) ) ;
#5638=ORIENTED_EDGE ( 'NONE', *, *, #7248, .F. ) ;
#5640=LINE ( 'NONE', #1739, #8400 ) ;
#5642=CARTESIAN_POINT ( 'NONE',  ( 136.6666666666666288, -15.00000000000000000, 159.8500000000001080 ) ) ;
#5669=CARTESIAN_POINT ( 'NONE',  ( 170.9999999999999716, -4.999999999999998224, 140.0000000000000000 ) ) ;
#5684=EDGE_LOOP ( 'NONE', ( #7918, #4597, #1023, #6893 ) ) ;
#5690=CARTESIAN_POINT ( 'NONE',  ( 303.3333333333333144, -15.00000000000000000, 162.5000000000000853 ) ) ;
#5694=VERTEX_POINT ( 'NONE', #2006 ) ;
#5698=VECTOR ( 'NONE', #8425, 1000.000000000000000 ) ;
#5710=CYLINDRICAL_SURFACE ( 'NONE', #6522, 2.649999999999985700 ) ;
#5722=EDGE_LOOP ( 'NONE', ( #5957, #5086, #2093, #8226 ) ) ;
#5724=EDGE_CURVE ( 'NONE', #3602, #4249, #6645, .T. ) ;
#5733=EDGE_LOOP ( 'NONE', ( #6701, #2750, #1680, #8428 ) ) ;
#5737=LINE ( 'NONE', #3788, #3105 ) ;
#5745=VERTEX_POINT ( 'NONE', #780 ) ;
#5752=LINE ( 'NONE', #6363, #5698 ) ;
#5755=VERTEX_POINT ( 'NONE', #2259 ) ;
#5764=DIRECTION ( 'NONE',  ( 1.000000000000000000, 0.000000000000000000, 0.000000000000000000 ) ) ;
#5772=VECTOR ( 'NONE', #3131, 1000.000000000000000 ) ;
#5777=EDGE_LOOP ( 'NONE', ( #6553, #347, #4787, #4381 ) ) ;
#5778=ORIENTED_EDGE ( 'NONE', *, *, #7415, .T. ) ;
#5779=VECTOR ( 'NONE', #1377, 1000.000000000000000 ) ;
#5781=AXIS2_PLACEMENT_3D ( 'NONE', #2691, #1465, #6679 ) ;
#5785=EDGE_CURVE ( 'NONE', #6409, #2056, #4255, .T. ) ;
#5786=VECTOR ( 'NONE', #7767, 1000.000000000000000 ) ;
#5796=CARTESIAN_POINT ( 'NONE',  ( -30.00000000000002842, -20.00000000000000000, 140.0000000000000000 ) ) ;
#5803=CARTESIAN_POINT ( 'NONE',  ( 53.33333333333330017, -15.00000000000000000, 165.1500000000000625 ) ) ;
#5804=VERTEX_POINT ( 'NONE', #1559 ) ;
#5810=ORIENTED_EDGE ( 'NONE', *, *, #5886, .F. ) ;
#5813=DIRECTION ( 'NONE',  ( -1.734723475976807587E-16, 1.000000000000000000, 0.000000000000000000 ) ) ;
#5818=LINE ( 'NONE', #8494, #1738 ) ;
#5820=DIRECTION ( 'NONE',  ( -0.000000000000000000, 1.000000000000000000, -0.000000000000000000 ) ) ;
#5825=VECTOR ( 'NONE', #1979, 1000.000000000000000 ) ;
#5826=LINE ( 'NONE', #7015, #7254 ) ;
#5828=EDGE_CURVE ( 'NONE', #2056, #7704, #3479, .T. ) ;
#5829=LINE ( 'NONE', #7887, #5786 ) ;
#5833=PLANE ( 'NONE',  #7245 ) ;
#5834=DIRECTION ( 'NONE',  ( 0.000000000000000000, 0.000000000000000000, 1.000000000000000000 ) ) ;
#5843=ORIENTED_EDGE ( 'NONE', *, *, #1654, .T. ) ;
#5849=LINE ( 'NONE', #2731, #5779 ) ;
#5851=ADVANCED_FACE ( 'NONE', ( #244 ), #287, .T. ) ;
#5863=CARTESIAN_POINT ( 'NONE',  ( 170.9999999999999716, 5.000000000000001776, 139.9990000000000236 ) ) ;
#5864=CIRCLE ( 'NONE', #4346, 2.649999999999985700 ) ;
#5865=ADVANCED_FACE ( 'NONE', ( #2444 ), #7705, .F. ) ;
#5868=ORIENTED_EDGE ( 'NONE', *, *, #249, .F. ) ;
#5873=AXIS2_PLACEMENT_3D ( 'NONE', #5047, #7796, #1050 ) ;
#5879=VECTOR ( 'NONE', #4895, 1000.000000000000000 ) ;
#5881=CARTESIAN_POINT ( 'NONE',  ( 357.0000000000000000, 5.000000000000000000, 139.9990000000000236 ) ) ;
#5886=EDGE_CURVE ( 'NONE', #730, #3075, #5640, .T. ) ;
#5893=CARTESIAN_POINT ( 'NONE',  ( 303.3333333333333144, -20.00000000000000000, 165.1500000000000625 ) ) ;
#5897=EDGE_LOOP ( 'NONE', ( #7029, #3070, #2636, #6898 ) ) ;
#5898=CARTESIAN_POINT ( 'NONE',  ( 82.99999999999998579, 5.000000000000001776, 145.0000000000000284 ) ) ;
#5904=DIRECTION ( 'NONE',  ( 0.000000000000000000, 0.000000000000000000, 1.000000000000000000 ) ) ;
#5952=ORIENTED_EDGE ( 'NONE', *, *, #1276, .T. ) ;
#5956=DIRECTION ( 'NONE',  ( 0.000000000000000000, 0.000000000000000000, 1.000000000000000000 ) ) ;
#5957=ORIENTED_EDGE ( 'NONE', *, *, #3938, .T. ) ;
#5958=CARTESIAN_POINT ( 'NONE',  ( 93.00000000000000000, -4.999999999999998224, 140.0000000000000000 ) ) ;
#5966=LINE ( 'NONE', #4665, #6977 ) ;
#5969=EDGE_CURVE ( 'NONE', #7555, #4028, #8356, .T. ) ;
#5981=CARTESIAN_POINT ( 'NONE',  ( 5.000000000000001776, -4.999999999999998224, 145.0000000000000284 ) ) ;
#5983=PLANE ( 'NONE',  #4216 ) ;
#5987=CARTESIAN_POINT ( 'NONE',  ( 53.33333333333330017, -14.99999999999999822, 159.8500000000001080 ) ) ;
#6016=EDGE_LOOP ( 'NONE', ( #7862, #5027, #5044, #413 ) ) ;
#6020=CARTESIAN_POINT ( 'NONE',  ( 219.9999999999999716, -15.00000000000000000, 159.8500000000001080 ) ) ;
#6024=VERTEX_POINT ( 'NONE', #679 ) ;
#6027=DIRECTION ( 'NONE',  ( 0.000000000000000000, 0.000000000000000000, 1.000000000000000000 ) ) ;
#6041=ORIENTED_EDGE ( 'NONE', *, *, #2025, .T. ) ;
#6045=AXIS2_PLACEMENT_3D ( 'NONE', #1520, #6951, #4827 ) ;
#6062=VERTEX_POINT ( 'NONE', #5893 ) ;
#6075=EDGE_CURVE ( 'NONE', #6478, #3075, #7949, .T. ) ;
#6082=ORIENTED_EDGE ( 'NONE', *, *, #5724, .F. ) ;
#6110=DIRECTION ( 'NONE',  ( -1.000000000000000000, 1.734723475976807587E-16, 0.000000000000000000 ) ) ;
#6111=CARTESIAN_POINT ( 'NONE',  ( -4.999999999999998224, -4.999999999999998224, 140.0000000000000000 ) ) ;
#6131=CARTESIAN_POINT ( 'NONE',  ( 386.6666666666666288, -14.99999999999999822, 159.8500000000001080 ) ) ;
#6134=FACE_BOUND ( 'NONE', #3468, .T. ) ;
#6135=PRODUCT_DEFINITION_SHAPE ( 'NONE', 'NONE',  #2614 ) ;
#6136=PLANE ( 'NONE',  #1854 ) ;
#6141=VECTOR ( 'NONE', #4782, 1000.000000000000000 ) ;
#6150=DIRECTION ( 'NONE',  ( -0.000000000000000000, -0.000000000000000000, 1.000000000000000000 ) ) ;
#6151=VECTOR ( 'NONE', #733, 1000.000000000000000 ) ;
#6153=AXIS2_PLACEMENT_3D ( 'NONE', #6255, #6734, #8186 ) ;
#6167=CARTESIAN_POINT ( 'NONE',  ( 82.99999999999998579, 5.000000000000001776, 145.0000000000000284 ) ) ;
#6168=AXIS2_PLACEMENT_3D ( 'NONE', #4045, #734, #4006 ) ;
#6169=CARTESIAN_POINT ( 'NONE',  ( -4.999999999999998224, -4.999999999999998224, 145.0000000000000284 ) ) ;
#6177=PLANE ( 'NONE',  #7546 ) ;
#6178=CARTESIAN_POINT ( 'NONE',  ( 347.0000000000000000, -4.999999999999998224, 145.0000000000000284 ) ) ;
#6180=DIRECTION ( 'NONE',  ( -0.000000000000000000, -0.000000000000000000, 1.000000000000000000 ) ) ;
#6186=VECTOR ( 'NONE', #4785, 1000.000000000000000 ) ;
#6188=DIRECTION ( 'NONE',  ( -1.734723475976807587E-16, 1.000000000000000000, 0.000000000000000000 ) ) ;
#6189=CARTESIAN_POINT ( 'NONE',  ( 444.9999999999999432, 5.000000000000000000, 139.9990000000000236 ) ) ;
#6210=EDGE_CURVE ( 'NONE', #819, #6781, #5502, .T. ) ;
#6213=DIRECTION ( 'NONE',  ( 0.000000000000000000, 0.000000000000000000, 1.000000000000000000 ) ) ;
#6215=LINE ( 'NONE', #4217, #5080 ) ;
#6217=ORIENTED_EDGE ( 'NONE', *, *, #3056, .T. ) ;
#6219=DIRECTION ( 'NONE',  ( 1.000000000000000000, 0.000000000000000000, -0.000000000000000000 ) ) ;
#6220=ORIENTED_EDGE ( 'NONE', *, *, #7528, .F. ) ;
#6227=FACE_BOUND ( 'NONE', #4004, .T. ) ;
#6243=VECTOR ( 'NONE', #2330, 1000.000000000000000 ) ;
#6244=EDGE_CURVE ( 'NONE', #7506, #6477, #3670, .T. ) ;
#6248=( LENGTH_UNIT ( ) NAMED_UNIT ( * ) SI_UNIT ( .MILLI., .METRE. ) );
#6251=EDGE_LOOP ( 'NONE', ( #4230, #6041, #4937, #6947 ) ) ;
#6255=CARTESIAN_POINT ( 'NONE',  ( 303.3333333333333144, -15.00000000000000000, 162.5000000000000853 ) ) ;
#6260=PLANE ( 'NONE',  #1120 ) ;
#6270=FACE_BOUND ( 'NONE', #6762, .T. ) ;
#6282=ORIENTED_EDGE ( 'NONE', *, *, #681, .F. ) ;
#6288=ORIENTED_EDGE ( 'NONE', *, *, #6908, .T. ) ;
#6290=VECTOR ( 'NONE', #1997, 1000.000000000000000 ) ;
#6292=DIRECTION ( 'NONE',  ( 0.000000000000000000, 0.000000000000000000, 1.000000000000000000 ) ) ;
#6294=ORIENTED_EDGE ( 'NONE', *, *, #7443, .T. ) ;
#6303=CIRCLE ( 'NONE', #5614, 2.649999999999985700 ) ;
#6330=AXIS2_PLACEMENT_3D ( 'NONE', #2577, #1797, #433 ) ;
#6337=DIRECTION ( 'NONE',  ( -0.000000000000000000, 1.000000000000000000, -0.000000000000000000 ) ) ;
#6339=VECTOR ( 'NONE', #859, 1000.000000000000000 ) ;
#6363=CARTESIAN_POINT ( 'NONE',  ( 434.9999999999999432, -4.999999999999998224, 145.0000000000000284 ) ) ;
#6367=EDGE_LOOP ( 'NONE', ( #6282, #4506, #3017, #861 ) ) ;
#6368=VECTOR ( 'NONE', #3098, 1000.000000000000000 ) ;
#6374=ORIENTED_EDGE ( 'NONE', *, *, #3565, .T. ) ;
#6386=CIRCLE ( 'NONE', #7358, 2.649999999999985700 ) ;
#6388=DIRECTION ( 'NONE',  ( 1.000000000000000000, 0.000000000000000000, 0.000000000000000000 ) ) ;
#6399=DIRECTION ( 'NONE',  ( 0.000000000000000000, 1.000000000000000000, 0.000000000000000000 ) ) ;
#6406=LINE ( 'NONE', #5796, #4996 ) ;
#6409=VERTEX_POINT ( 'NONE', #2342 ) ;
#6412=CARTESIAN_POINT ( 'NONE',  ( 269.0000000000000000, 5.000000000000000000, 140.0000000000000000 ) ) ;
#6415=APPLICATION_CONTEXT ( 'automotive_design' ) ;
#6421=( LENGTH_UNIT ( ) NAMED_UNIT ( * ) SI_UNIT ( .MILLI., .METRE. ) );
#6429=EDGE_CURVE ( 'NONE', #5755, #8497, #1067, .T. ) ;
#6432=CARTESIAN_POINT ( 'NONE',  ( 170.9999999999999716, -4.999999999999998224, 145.0000000000000284 ) ) ;
#6433=ORIENTED_EDGE ( 'NONE', *, *, #67, .F. ) ;
#6445=CARTESIAN_POINT ( 'NONE',  ( 269.0000000000000000, -4.999999999999998224, 139.9990000000000236 ) ) ;
#6452=DIRECTION ( 'NONE',  ( 0.000000000000000000, -1.000000000000000000, 0.000000000000000000 ) ) ;
#6453=DIRECTION ( 'NONE',  ( -0.000000000000000000, 1.000000000000000000, -0.000000000000000000 ) ) ;
#6454=DIRECTION ( 'NONE',  ( 0.000000000000000000, 0.000000000000000000, 1.000000000000000000 ) ) ;
#6458=CARTESIAN_POINT ( 'NONE',  ( 303.3333333333333144, -14.99999999999999822, 162.5000000000000853 ) ) ;
#6463=CARTESIAN_POINT ( 'NONE',  ( -30.00000000000000000, 15.00000000000000000, 145.0000000000000284 ) ) ;
#6476=CARTESIAN_POINT ( 'NONE',  ( 181.0000000000000000, -4.999999999999998224, 140.0000000000000000 ) ) ;
#6477=VERTEX_POINT ( 'NONE', #3326 ) ;
#6478=VERTEX_POINT ( 'NONE', #7856 ) ;
#6481=VECTOR ( 'NONE', #6110, 1000.000000000000000 ) ;
#6503=EDGE_CURVE ( 'NONE', #3186, #8497, #6303, .T. ) ;
#6507=ORIENTED_EDGE ( 'NONE', *, *, #6764, .F. ) ;
#6510=CARTESIAN_POINT ( 'NONE',  ( 5.000000000000001776, -4.999999999999998224, 139.9990000000000236 ) ) ;
#6522=AXIS2_PLACEMENT_3D ( 'NONE', #8382, #6453, #5060 ) ;
#6523=FACE_OUTER_BOUND ( 'NONE', #6367, .T. ) ;
#6532=CARTESIAN_POINT ( 'NONE',  ( 347.0000000000000000, -4.999999999999998224, 140.0000000000000000 ) ) ;
#6553=ORIENTED_EDGE ( 'NONE', *, *, #6210, .T. ) ;
#6554=MECHANICAL_DESIGN_GEOMETRIC_PRESENTATION_REPRESENTATION('',(#581),#4753);
#6564=VERTEX_POINT ( 'NONE', #8597 ) ;
#6565=EDGE_CURVE ( 'NONE', #8255, #6478, #3242, .T. ) ;
#6568=VERTEX_POINT ( 'NONE', #5232 ) ;
#6589=ORIENTED_EDGE ( 'NONE', *, *, #8432, .F. ) ;
#6593=DIRECTION ( 'NONE',  ( 1.734723475976807587E-16, 1.000000000000000000, 0.000000000000000000 ) ) ;
#6595=ORIENTED_EDGE ( 'NONE', *, *, #234, .F. ) ;
#6602=DIRECTION ( 'NONE',  ( 0.000000000000000000, 0.000000000000000000, 1.000000000000000000 ) ) ;
#6615=CYLINDRICAL_SURFACE ( 'NONE', #3049, 2.649999999999985700 ) ;
#6616=ORIENTED_EDGE ( 'NONE', *, *, #3379, .F. ) ;
#6619=VECTOR ( 'NONE', #2427, 1000.000000000000000 ) ;
#6620=VECTOR ( 'NONE', #8560, 1000.000000000000000 ) ;
#6624=DIRECTION ( 'NONE',  ( -0.000000000000000000, -1.000000000000000000, -0.000000000000000000 ) ) ;
#6630=EDGE_LOOP ( 'NONE', ( #786, #640, #991, #6589 ) ) ;
#6636=EDGE_CURVE ( 'NONE', #4134, #5482, #6876, .T. ) ;
#6643=ORIENTED_EDGE ( 'NONE', *, *, #5606, .F. ) ;
#6645=LINE ( 'NONE', #691, #6714 ) ;
#6649=VECTOR ( 'NONE', #2400, 1000.000000000000000 ) ;
#6666=CARTESIAN_POINT ( 'NONE',  ( 136.6666666666666288, -20.00000000000000000, 159.8500000000001080 ) ) ;
#6669=EDGE_CURVE ( 'NONE', #8497, #3186, #6727, .T. ) ;
#6679=DIRECTION ( 'NONE',  ( 0.000000000000000000, 0.000000000000000000, 1.000000000000000000 ) ) ;
#6686=LINE ( 'NONE', #4517, #6151 ) ;
#6691=CYLINDRICAL_SURFACE ( 'NONE', #4012, 2.649999999999985700 ) ;
#6700=CARTESIAN_POINT ( 'NONE',  ( 386.6666666666666288, -15.00000000000000000, 162.5000000000000853 ) ) ;
#6701=ORIENTED_EDGE ( 'NONE', *, *, #1949, .T. ) ;
#6713=ORIENTED_EDGE ( 'NONE', *, *, #1847, .F. ) ;
#6714=VECTOR ( 'NONE', #4692, 1000.000000000000000 ) ;
#6716=EDGE_CURVE ( 'NONE', #5045, #5286, #3531, .T. ) ;
#6721=VECTOR ( 'NONE', #162, 1000.000000000000000 ) ;
#6727=CIRCLE ( 'NONE', #2988, 2.649999999999985700 ) ;
#6728=LINE ( 'NONE', #18, #6339 ) ;
#6732=ORIENTED_EDGE ( 'NONE', *, *, #7280, .T. ) ;
#6734=DIRECTION ( 'NONE',  ( -0.000000000000000000, 1.000000000000000000, -0.000000000000000000 ) ) ;
#6750=EDGE_CURVE ( 'NONE', #2735, #3700, #2672, .T. ) ;
#6758=LINE ( 'NONE', #2849, #4126 ) ;
#6762=EDGE_LOOP ( 'NONE', ( #1331, #8310 ) ) ;
#6764=EDGE_CURVE ( 'NONE', #5482, #3613, #5818, .T. ) ;
#6771=LINE ( 'NONE', #3473, #6481 ) ;
#6773=( NAMED_UNIT ( * ) PLANE_ANGLE_UNIT ( ) SI_UNIT ( $, .RADIAN. ) );
#6776=ORIENTED_EDGE ( 'NONE', *, *, #580, .T. ) ;
#6781=VERTEX_POINT ( 'NONE', #3094 ) ;
#6790=FACE_BOUND ( 'NONE', #3137, .T. ) ;
#6794=DIRECTION ( 'NONE',  ( -0.000000000000000000, 1.000000000000000000, -0.000000000000000000 ) ) ;
#6807=ADVANCED_FACE ( 'NONE', ( #3140 ), #7006, .F. ) ;
#6821=CARTESIAN_POINT ( 'NONE',  ( 269.0000000000000000, -4.999999999999998224, 139.9990000000000236 ) ) ;
#6823=ORIENTED_EDGE ( 'NONE', *, *, #5078, .T. ) ;
#6829=EDGE_CURVE ( 'NONE', #6564, #1248, #7759, .T. ) ;
#6839=FACE_OUTER_BOUND ( 'NONE', #5684, .T. ) ;
#6876=LINE ( 'NONE', #4312, #6721 ) ;
#6879=DIRECTION ( 'NONE',  ( 0.000000000000000000, 0.000000000000000000, 1.000000000000000000 ) ) ;
#6883=CARTESIAN_POINT ( 'NONE',  ( 470.0000000000000000, 15.00000000000000000, 145.0000000000000284 ) ) ;
#6893=ORIENTED_EDGE ( 'NONE', *, *, #2002, .T. ) ;
#6896=DIRECTION ( 'NONE',  ( 1.000000000000000000, 0.000000000000000000, 0.000000000000000000 ) ) ;
#6898=ORIENTED_EDGE ( 'NONE', *, *, #4396, .F. ) ;
#6908=EDGE_CURVE ( 'NONE', #3700, #1248, #388, .T. ) ;
#6910=ADVANCED_FACE ( 'NONE', ( #3180 ), #7137, .F. ) ;
#6913=ORIENTED_EDGE ( 'NONE', *, *, #201, .T. ) ;
#6923=DIRECTION ( 'NONE',  ( -0.000000000000000000, -0.000000000000000000, 1.000000000000000000 ) ) ;
#6928=ADVANCED_FACE ( 'NONE', ( #606 ), #2007, .F. ) ;
#6939=EDGE_CURVE ( 'NONE', #6477, #7506, #5475, .T. ) ;
#6942=EDGE_LOOP ( 'NONE', ( #3572, #1545, #2046, #7613 ) ) ;
#6943=FILL_AREA_STYLE ('',( #4382 ) ) ;
#6944=CARTESIAN_POINT ( 'NONE',  ( 136.6666666666666288, -14.99999999999999822, 162.5000000000000853 ) ) ;
#6947=ORIENTED_EDGE ( 'NONE', *, *, #2375, .F. ) ;
#6951=DIRECTION ( 'NONE',  ( 0.000000000000000000, 1.000000000000000000, 0.000000000000000000 ) ) ;
#6953=ORIENTED_EDGE ( 'NONE', *, *, #1892, .T. ) ;
#6971=CARTESIAN_POINT ( 'NONE',  ( 136.6666666666666288, -20.00000000000000000, 162.5000000000000853 ) ) ;
#6974=VECTOR ( 'NONE', #1466, 1000.000000000000000 ) ;
#6975=ORIENTED_EDGE ( 'NONE', *, *, #4059, .F. ) ;
#6977=VECTOR ( 'NONE', #6624, 1000.000000000000000 ) ;
#6983=AXIS2_PLACEMENT_3D ( 'NONE', #3571, #6219, #8235 ) ;
#6985=EDGE_LOOP ( 'NONE', ( #3785, #318 ) ) ;
#6987=DIRECTION ( 'NONE',  ( 0.000000000000000000, 0.000000000000000000, 1.000000000000000000 ) ) ;
#6988=EDGE_CURVE ( 'NONE', #1439, #54, #7284, .T. ) ;
#6998=FACE_OUTER_BOUND ( 'NONE', #656, .T. ) ;
#7002=FACE_OUTER_BOUND ( 'NONE', #3462, .T. ) ;
#7006=PLANE ( 'NONE',  #3258 ) ;
#7011=VERTEX_POINT ( 'NONE', #5387 ) ;
#7015=CARTESIAN_POINT ( 'NONE',  ( -30.00000000000000000, -15.00000000000000000, 140.0000000000000000 ) ) ;
#7020=ADVANCED_FACE ( 'NONE', ( #7351 ), #1340, .F. ) ;
#7029=ORIENTED_EDGE ( 'NONE', *, *, #4759, .F. ) ;
#7032=ORIENTED_EDGE ( 'NONE', *, *, #4396, .T. ) ;
#7036=ORIENTED_EDGE ( 'NONE', *, *, #6503, .F. ) ;
#7056=VERTEX_POINT ( 'NONE', #26 ) ;
#7060=LINE ( 'NONE', #5669, #7509 ) ;
#7064=EDGE_CURVE ( 'NONE', #54, #1439, #3959, .T. ) ;
#7067=EDGE_CURVE ( 'NONE', #2451, #1549, #245, .T. ) ;
#7077=ORIENTED_EDGE ( 'NONE', *, *, #1575, .T. ) ;
#7082=DIRECTION ( 'NONE',  ( 0.000000000000000000, -1.000000000000000000, 0.000000000000000000 ) ) ;
#7105=ORIENTED_EDGE ( 'NONE', *, *, #7723, .T. ) ;
#7120=ORIENTED_EDGE ( 'NONE', *, *, #7318, .F. ) ;
#7126=EDGE_CURVE ( 'NONE', #8255, #730, #955, .T. ) ;
#7127=LINE ( 'NONE', #473, #3145 ) ;
#7131=DIRECTION ( 'NONE',  ( -1.000000000000000000, 0.000000000000000000, -0.000000000000000000 ) ) ;
#7133=VECTOR ( 'NONE', #5034, 1000.000000000000000 ) ;
#7136=DIRECTION ( 'NONE',  ( -1.734723475976807587E-16, 1.000000000000000000, 0.000000000000000000 ) ) ;
#7137=PLANE ( 'NONE',  #331 ) ;
#7138=AXIS2_PLACEMENT_3D ( 'NONE', #5374, #8046, #2077 ) ;
#7148=ADVANCED_FACE ( 'NONE', ( #911 ), #4256, .F. ) ;
#7157=DIRECTION ( 'NONE',  ( -0.000000000000000000, 1.000000000000000000, -0.000000000000000000 ) ) ;
#7158=CARTESIAN_POINT ( 'NONE',  ( 170.9999999999999716, -4.999999999999998224, 145.0000000000000284 ) ) ;
#7166=DIRECTION ( 'NONE',  ( 0.000000000000000000, -0.000000000000000000, -1.000000000000000000 ) ) ;
#7167=ORIENTED_EDGE ( 'NONE', *, *, #1149, .F. ) ;
#7186=VERTEX_POINT ( 'NONE', #3520 ) ;
#7188=DIRECTION ( 'NONE',  ( -1.000000000000000000, 1.734723475976807341E-16, -0.000000000000000000 ) ) ;
#7212=ORIENTED_EDGE ( 'NONE', *, *, #4173, .F. ) ;
#7213=VERTEX_POINT ( 'NONE', #289 ) ;
#7219=CARTESIAN_POINT ( 'NONE',  ( 269.0000000000000000, 5.000000000000000000, 145.0000000000000284 ) ) ;
#7220=VERTEX_POINT ( 'NONE', #6167 ) ;
#7223=DIRECTION ( 'NONE',  ( -1.000000000000000000, 1.734723475976807341E-16, -0.000000000000000000 ) ) ;
#7227=CARTESIAN_POINT ( 'NONE',  ( -4.999999999999998224, 5.000000000000001776, 145.0000000000000284 ) ) ;
#7238=LINE ( 'NONE', #5803, #6620 ) ;
#7240=ORIENTED_EDGE ( 'NONE', *, *, #6829, .T. ) ;
#7245=AXIS2_PLACEMENT_3D ( 'NONE', #8507, #1896, #7566 ) ;
#7248=EDGE_CURVE ( 'NONE', #2875, #2638, #3130, .T. ) ;
#7250=CARTESIAN_POINT ( 'NONE',  ( 303.3333333333333144, -14.99999999999999822, 159.8500000000001080 ) ) ;
#7254=VECTOR ( 'NONE', #5260, 1000.000000000000000 ) ;
#7262=CARTESIAN_POINT ( 'NONE',  ( 5.000000000000001776, -4.999999999999998224, 139.9990000000000236 ) ) ;
#7278=LINE ( 'NONE', #5313, #2260 ) ;
#7280=EDGE_CURVE ( 'NONE', #1907, #4164, #8483, .T. ) ;
#7284=CIRCLE ( 'NONE', #8548, 2.649999999999985700 ) ;
#7296=ORIENTED_EDGE ( 'NONE', *, *, #7720, .T. ) ;
#7309=FACE_OUTER_BOUND ( 'NONE', #8355, .T. ) ;
#7316=VECTOR ( 'NONE', #324, 1000.000000000000000 ) ;
#7318=EDGE_CURVE ( 'NONE', #5694, #238, #3045, .T. ) ;
#7329=DIRECTION ( 'NONE',  ( 1.000000000000000000, 0.000000000000000000, 0.000000000000000000 ) ) ;
#7342=EDGE_LOOP ( 'NONE', ( #675, #1054, #1621, #3718 ) ) ;
#7344=FACE_OUTER_BOUND ( 'NONE', #715, .T. ) ;
#7351=FACE_OUTER_BOUND ( 'NONE', #169, .T. ) ;
#7358=AXIS2_PLACEMENT_3D ( 'NONE', #6971, #5576, #5537 ) ;
#7371=DIRECTION ( 'NONE',  ( 0.000000000000000000, 0.000000000000000000, 1.000000000000000000 ) ) ;
#7384=DIRECTION ( 'NONE',  ( -1.000000000000000000, 1.734723475976807587E-16, 0.000000000000000000 ) ) ;
#7387=ORIENTED_EDGE ( 'NONE', *, *, #5078, .F. ) ;
#7390=DIRECTION ( 'NONE',  ( -0.000000000000000000, 1.000000000000000000, -0.000000000000000000 ) ) ;
#7391=DIRECTION ( 'NONE',  ( 1.000000000000000000, 0.000000000000000000, 0.000000000000000000 ) ) ;
#7413=ADVANCED_FACE ( 'NONE', ( #1208 ), #2685, .F. ) ;
#7414=CARTESIAN_POINT ( 'NONE',  ( 386.6666666666666288, -20.00000000000000000, 165.1500000000000625 ) ) ;
#7415=EDGE_CURVE ( 'NONE', #819, #1874, #7908, .T. ) ;
#7419=ORIENTED_EDGE ( 'NONE', *, *, #7800, .T. ) ;
#7431=LINE ( 'NONE', #4163, #7688 ) ;
#7433=ORIENTED_EDGE ( 'NONE', *, *, #4360, .F. ) ;
#7438=ORIENTED_EDGE ( 'NONE', *, *, #1375, .T. ) ;
#7443=EDGE_CURVE ( 'NONE', #5265, #58, #1950, .T. ) ;
#7447=CARTESIAN_POINT ( 'NONE',  ( 93.00000000000000000, 5.000000000000000000, 139.9990000000000236 ) ) ;
#7452=VECTOR ( 'NONE', #3469, 1000.000000000000000 ) ;
#7457=CARTESIAN_POINT ( 'NONE',  ( -30.00000000000002842, -15.00000000000000000, 180.0000000000000284 ) ) ;
#7458=AXIS2_PLACEMENT_3D ( 'NONE', #3663, #2968, #5486 ) ;
#7467=EDGE_CURVE ( 'NONE', #6024, #874, #3292, .T. ) ;
#7471=DIRECTION ( 'NONE',  ( 0.000000000000000000, 1.000000000000000000, 0.000000000000000000 ) ) ;
#7493=FACE_OUTER_BOUND ( 'NONE', #6942, .T. ) ;
#7500=VECTOR ( 'NONE', #6188, 1000.000000000000000 ) ;
#7506=VERTEX_POINT ( 'NONE', #1286 ) ;
#7509=VECTOR ( 'NONE', #6452, 1000.000000000000000 ) ;
#7528=EDGE_CURVE ( 'NONE', #3247, #7506, #680, .T. ) ;
#7530=ORIENTED_EDGE ( 'NONE', *, *, #4807, .F. ) ;
#7537=ORIENTED_EDGE ( 'NONE', *, *, #6669, .F. ) ;
#7538=FACE_BOUND ( 'NONE', #4349, .T. ) ;
#7541=AXIS2_PLACEMENT_3D ( 'NONE', #4365, #5096, #1802 ) ;
#7546=AXIS2_PLACEMENT_3D ( 'NONE', #920, #255, #5564 ) ;
#7555=VERTEX_POINT ( 'NONE', #1547 ) ;
#7564=DIRECTION ( 'NONE',  ( 0.000000000000000000, -0.000000000000000000, -1.000000000000000000 ) ) ;
#7566=DIRECTION ( 'NONE',  ( -1.000000000000000000, 1.734723475976807587E-16, 0.000000000000000000 ) ) ;
#7571=EDGE_CURVE ( 'NONE', #6564, #5265, #8218, .T. ) ;
#7582=DIRECTION ( 'NONE',  ( 1.000000000000000000, 0.000000000000000000, 0.000000000000000000 ) ) ;
#7585=PLANE ( 'NONE',  #3316 ) ;
#7591=ADVANCED_FACE ( 'NONE', ( #2727 ), #2160, .F. ) ;
#7593=CARTESIAN_POINT ( 'NONE',  ( 444.9999999999999432, -4.999999999999998224, 140.0000000000000000 ) ) ;
#7595=CARTESIAN_POINT ( 'NONE',  ( 136.6666666666666288, -14.99999999999999822, 159.8500000000001080 ) ) ;
#7599=ORIENTED_EDGE ( 'NONE', *, *, #7467, .F. ) ;
#7606=AXIS2_PLACEMENT_3D ( 'NONE', #2713, #796, #6879 ) ;
#7609=VERTEX_POINT ( 'NONE', #2987 ) ;
#7613=ORIENTED_EDGE ( 'NONE', *, *, #249, .T. ) ;
#7618=LINE ( 'NONE', #4997, #6649 ) ;
#7623=ORIENTED_EDGE ( 'NONE', *, *, #6716, .F. ) ;
#7632=ORIENTED_EDGE ( 'NONE', *, *, #3565, .F. ) ;
#7633=DIRECTION ( 'NONE',  ( -1.000000000000000000, 1.734723475976807587E-16, 0.000000000000000000 ) ) ;
#7638=CARTESIAN_POINT ( 'NONE',  ( 357.0000000000000000, -4.999999999999998224, 140.0000000000000000 ) ) ;
#7654=DIRECTION ( 'NONE',  ( -0.000000000000000000, 1.000000000000000000, -0.000000000000000000 ) ) ;
#7655=EDGE_LOOP ( 'NONE', ( #5245, #1799 ) ) ;
#7668=EDGE_CURVE ( 'NONE', #5265, #7722, #1682, .T. ) ;
#7673=PLANE ( 'NONE',  #4944 ) ;
#7675=CARTESIAN_POINT ( 'NONE',  ( -30.00000000000000000, 15.00000000000000000, 140.0000000000000000 ) ) ;
#7687=ORIENTED_EDGE ( 'NONE', *, *, #6750, .T. ) ;
#7688=VECTOR ( 'NONE', #729, 1000.000000000000000 ) ;
#7692=CARTESIAN_POINT ( 'NONE',  ( 5.000000000000000000, 5.000000000000000000, 140.0000000000000000 ) ) ;
#7696=EDGE_CURVE ( 'NONE', #5804, #6568, #4288, .T. ) ;
#7700=AXIS2_PLACEMENT_3D ( 'NONE', #8274, #993, #4340 ) ;
#7703=AXIS2_PLACEMENT_3D ( 'NONE', #522, #3833, #7136 ) ;
#7704=VERTEX_POINT ( 'NONE', #8389 ) ;
#7705=PLANE ( 'NONE',  #3522 ) ;
#7710=ORIENTED_EDGE ( 'NONE', *, *, #7280, .F. ) ;
#7720=EDGE_CURVE ( 'NONE', #1874, #5745, #2938, .T. ) ;
#7722=VERTEX_POINT ( 'NONE', #7692 ) ;
#7723=EDGE_CURVE ( 'NONE', #7722, #2735, #1638, .T. ) ;
#7734=AXIS2_PLACEMENT_3D ( 'NONE', #4695, #1390, #4046 ) ;
#7741=SURFACE_STYLE_USAGE ( .BOTH. , #8399 ) ;
#7748=CIRCLE ( 'NONE', #5092, 2.649999999999985700 ) ;
#7757=ORIENTED_EDGE ( 'NONE', *, *, #3348, .F. ) ;
#7759=LINE ( 'NONE', #1881, #7848 ) ;
#7762=ORIENTED_EDGE ( 'NONE', *, *, #1263, .F. ) ;
#7763=ORIENTED_EDGE ( 'NONE', *, *, #580, .F. ) ;
#7767=DIRECTION ( 'NONE',  ( -0.000000000000000000, -0.000000000000000000, 1.000000000000000000 ) ) ;
#7775=CARTESIAN_POINT ( 'NONE',  ( 434.9999999999999432, -4.999999999999998224, 139.9990000000000236 ) ) ;
#7779=ORIENTED_EDGE ( 'NONE', *, *, #5969, .T. ) ;
#7782=ORIENTED_EDGE ( 'NONE', *, *, #1213, .F. ) ;
#7790=EDGE_CURVE ( 'NONE', #4735, #3602, #5966, .T. ) ;
#7792=LINE ( 'NONE', #427, #8217 ) ;
#7793=ORIENTED_EDGE ( 'NONE', *, *, #849, .T. ) ;
#7796=DIRECTION ( 'NONE',  ( -0.000000000000000000, 1.000000000000000000, -0.000000000000000000 ) ) ;
#7799=EDGE_CURVE ( 'NONE', #716, #5045, #2513, .T. ) ;
#7800=EDGE_CURVE ( 'NONE', #5335, #1123, #3982, .T. ) ;
#7802=LINE ( 'NONE', #2367, #6368 ) ;
#7810=CARTESIAN_POINT ( 'NONE',  ( 434.9999999999999432, -4.999999999999998224, 145.0000000000000284 ) ) ;
#7826=VECTOR ( 'NONE', #705, 1000.000000000000000 ) ;
#7829=ORIENTED_EDGE ( 'NONE', *, *, #1375, .F. ) ;
#7844=CARTESIAN_POINT ( 'NONE',  ( 136.6666666666666288, -15.00000000000000000, 162.5000000000000853 ) ) ;
#7848=VECTOR ( 'NONE', #8327, 1000.000000000000000 ) ;
#7849=LINE ( 'NONE', #3803, #3713 ) ;
#7855=EDGE_CURVE ( 'NONE', #8118, #186, #1318, .T. ) ;
#7856=CARTESIAN_POINT ( 'NONE',  ( 357.0000000000000000, 5.000000000000000000, 145.0000000000000284 ) ) ;
#7862=ORIENTED_EDGE ( 'NONE', *, *, #6750, .F. ) ;
#7870=DIRECTION ( 'NONE',  ( 1.000000000000000000, 0.000000000000000000, 0.000000000000000000 ) ) ;
#7873=EDGE_LOOP ( 'NONE', ( #5416, #6776, #4460, #3988 ) ) ;
#7881=VECTOR ( 'NONE', #7223, 1000.000000000000000 ) ;
#7887=CARTESIAN_POINT ( 'NONE',  ( 259.0000000000000000, 5.000000000000001776, 139.9990000000000236 ) ) ;
#7908=LINE ( 'NONE', #3866, #4490 ) ;
#7918=ORIENTED_EDGE ( 'NONE', *, *, #4897, .T. ) ;
#7924=LINE ( 'NONE', #31, #2365 ) ;
#7942=LINE ( 'NONE', #5406, #5825 ) ;
#7949=LINE ( 'NONE', #545, #48 ) ;
#7957=LINE ( 'NONE', #553, #6290 ) ;
#7960=EDGE_CURVE ( 'NONE', #3209, #4134, #1449, .T. ) ;
#7962=CYLINDRICAL_SURFACE ( 'NONE', #3091, 2.649999999999985700 ) ;
#7965=ORIENTED_EDGE ( 'NONE', *, *, #7126, .F. ) ;
#7986=DIRECTION ( 'NONE',  ( -1.734723475976807341E-16, 1.000000000000000000, 0.000000000000000000 ) ) ;
#7988=CARTESIAN_POINT ( 'NONE',  ( 347.0000000000000000, -4.999999999999998224, 139.9990000000000236 ) ) ;
#7993=SHAPE_REPRESENTATION ( 'side rail', ( #594 ), #2832 ) ;
#7994=EDGE_LOOP ( 'NONE', ( #4056, #3859 ) ) ;
#8002=ORIENTED_EDGE ( 'NONE', *, *, #3808, .F. ) ;
#8009=ORIENTED_EDGE ( 'NONE', *, *, #7696, .F. ) ;
#8015=VECTOR ( 'NONE', #5032, 1000.000000000000000 ) ;
#8018=DIRECTION ( 'NONE',  ( -0.000000000000000000, 1.000000000000000000, -0.000000000000000000 ) ) ;
#8031=CIRCLE ( 'NONE', #3575, 2.649999999999985700 ) ;
#8036=DIRECTION ( 'NONE',  ( 1.000000000000000000, 0.000000000000000000, 0.000000000000000000 ) ) ;
#8040=EDGE_LOOP ( 'NONE', ( #6595, #5478 ) ) ;
#8041=EDGE_LOOP ( 'NONE', ( #611, #3048, #6217, #1507 ) ) ;
#8046=DIRECTION ( 'NONE',  ( 1.734723475976807587E-16, 1.000000000000000000, 0.000000000000000000 ) ) ;
#8054=ORIENTED_EDGE ( 'NONE', *, *, #2628, .F. ) ;
#8082=LINE ( 'NONE', #182, #5365 ) ;
#8093=ORIENTED_EDGE ( 'NONE', *, *, #5606, .T. ) ;
#8100=CARTESIAN_POINT ( 'NONE',  ( 53.33333333333330017, -14.99999999999999822, 162.5000000000000853 ) ) ;
#8112=ORIENTED_EDGE ( 'NONE', *, *, #5397, .F. ) ;
#8118=VERTEX_POINT ( 'NONE', #7593 ) ;
#8119=FACE_BOUND ( 'NONE', #4037, .T. ) ;
#8125=LINE ( 'NONE', #763, #2771 ) ;
#8139=DIRECTION ( 'NONE',  ( 1.734723475976807587E-16, 1.000000000000000000, 0.000000000000000000 ) ) ;
#8140=DIRECTION ( 'NONE',  ( -0.000000000000000000, 1.000000000000000000, -0.000000000000000000 ) ) ;
#8146=LINE ( 'NONE', #1472, #3161 ) ;
#8159=FACE_OUTER_BOUND ( 'NONE', #2795, .T. ) ;
#8178=CARTESIAN_POINT ( 'NONE',  ( 170.9999999999999716, -4.999999999999998224, 139.9990000000000236 ) ) ;
#8183=ORIENTED_EDGE ( 'NONE', *, *, #5522, .T. ) ;
#8186=DIRECTION ( 'NONE',  ( 0.000000000000000000, 0.000000000000000000, 1.000000000000000000 ) ) ;
#8190=VECTOR ( 'NONE', #8242, 1000.000000000000000 ) ;
#8194=ORIENTED_EDGE ( 'NONE', *, *, #1276, .F. ) ;
#8197=AXIS2_PLACEMENT_3D ( 'NONE', #957, #785, #5477 ) ;
#8205=DIRECTION ( 'NONE',  ( 0.000000000000000000, 0.000000000000000000, 1.000000000000000000 ) ) ;
#8213=ORIENTED_EDGE ( 'NONE', *, *, #2628, .T. ) ;
#8217=VECTOR ( 'NONE', #3652, 1000.000000000000000 ) ;
#8218=LINE ( 'NONE', #2855, #8532 ) ;
#8226=ORIENTED_EDGE ( 'NONE', *, *, #7960, .F. ) ;
#8235=DIRECTION ( 'NONE',  ( -0.000000000000000000, 0.000000000000000000, -1.000000000000000000 ) ) ;
#8239=CARTESIAN_POINT ( 'NONE',  ( 303.3333333333333144, -14.99999999999999822, 162.5000000000000853 ) ) ;
#8242=DIRECTION ( 'NONE',  ( -0.000000000000000000, -1.000000000000000000, -0.000000000000000000 ) ) ;
#8251=CARTESIAN_POINT ( 'NONE',  ( 170.9999999999999716, 5.000000000000001776, 139.9990000000000236 ) ) ;
#8253=DIRECTION ( 'NONE',  ( -0.000000000000000000, -0.000000000000000000, 1.000000000000000000 ) ) ;
#8255=VERTEX_POINT ( 'NONE', #4875 ) ;
#8259=EDGE_LOOP ( 'NONE', ( #6823, #6288, #1737, #2901 ) ) ;
#8261=DIRECTION ( 'NONE',  ( -0.000000000000000000, -0.000000000000000000, 1.000000000000000000 ) ) ;
#8263=VECTOR ( 'NONE', #3764, 1000.000000000000000 ) ;
#8274=CARTESIAN_POINT ( 'NONE',  ( -30.00000000000000000, -15.00000000000000000, 145.0000000000000284 ) ) ;
#8277=PLANE ( 'NONE',  #6045 ) ;
#8290=EDGE_LOOP ( 'NONE', ( #8398, #8112 ) ) ;
#8301=AXIS2_PLACEMENT_3D ( 'NONE', #2162, #4815, #902 ) ;
#8302=ORIENTED_EDGE ( 'NONE', *, *, #5570, .F. ) ;
#8309=EDGE_LOOP ( 'NONE', ( #4632, #2450, #8002, #2047 ) ) ;
#8310=ORIENTED_EDGE ( 'NONE', *, *, #7064, .T. ) ;
#8311=DIRECTION ( 'NONE',  ( 0.000000000000000000, 1.000000000000000000, 0.000000000000000000 ) ) ;
#8313=EDGE_LOOP ( 'NONE', ( #1475, #7032, #7212, #5638 ) ) ;
#8325=LINE ( 'NONE', #2363, #3517 ) ;
#8327=DIRECTION ( 'NONE',  ( -0.000000000000000000, -0.000000000000000000, 1.000000000000000000 ) ) ;
#8332=PLANE ( 'NONE',  #2641 ) ;
#8350=( NAMED_UNIT ( * ) SI_UNIT ( $, .STERADIAN. ) SOLID_ANGLE_UNIT ( ) );
#8355=EDGE_LOOP ( 'NONE', ( #6616, #6732, #4098, #4814 ) ) ;
#8356=LINE ( 'NONE', #2397, #8015 ) ;
#8358=ADVANCED_FACE ( 'NONE', ( #3401 ), #3443, .T. ) ;
#8368=CARTESIAN_POINT ( 'NONE',  ( 93.00000000000000000, -4.999999999999998224, 139.9990000000000236 ) ) ;
#8382=CARTESIAN_POINT ( 'NONE',  ( 219.9999999999999716, -15.00000000000000000, 162.5000000000000853 ) ) ;
#8387=CARTESIAN_POINT ( 'NONE',  ( 303.3333333333333144, -15.00000000000000000, 159.8500000000001080 ) ) ;
#8389=CARTESIAN_POINT ( 'NONE',  ( 470.0000000000000000, -15.00000000000000000, 180.0000000000000284 ) ) ;
#8393=CIRCLE ( 'NONE', #5873, 2.649999999999985700 ) ;
#8398=ORIENTED_EDGE ( 'NONE', *, *, #3272, .F. ) ;
#8399=SURFACE_SIDE_STYLE ('',( #416 ) ) ;
#8400=VECTOR ( 'NONE', #2996, 1000.000000000000000 ) ;
#8409=EDGE_CURVE ( 'NONE', #3613, #7220, #4685, .T. ) ;
#8414=FACE_OUTER_BOUND ( 'NONE', #1879, .T. ) ;
#8416=AXIS2_PLACEMENT_3D ( 'NONE', #5345, #1519, #6213 ) ;
#8418=FACE_OUTER_BOUND ( 'NONE', #1929, .T. ) ;
#8425=DIRECTION ( 'NONE',  ( -0.000000000000000000, -1.000000000000000000, -0.000000000000000000 ) ) ;
#8428=ORIENTED_EDGE ( 'NONE', *, *, #60, .F. ) ;
#8432=EDGE_CURVE ( 'NONE', #4191, #5694, #7957, .T. ) ;
#8438=ORIENTED_EDGE ( 'NONE', *, *, #7960, .T. ) ;
#8448=CLOSED_SHELL ( 'NONE', ( #3754, #2845, #3564, #3083, #3042, #167, #753, #1341, #5533, #5865, #6928, #5395, #4459, #7591, #2560, #1699, #986, #7413, #3834, #2758, #7020, #8358, #1152, #5851, #4536, #3720, #2630, #4993, #3766, #1048, #361, #5073, #4730, #6807, #6910, #87, #1129, #2455, #7148, #4591, #984, #1010 ) ) ;
#8464=LINE ( 'NONE', #1014, #5450 ) ;
#8470=DIRECTION ( 'NONE',  ( 1.000000000000000000, 0.000000000000000000, 0.000000000000000000 ) ) ;
#8476=EDGE_CURVE ( 'NONE', #6409, #6568, #3214, .T. ) ;
#8483=LINE ( 'NONE', #5642, #3800 ) ;
#8494=CARTESIAN_POINT ( 'NONE',  ( 93.00000000000000000, -4.999999999999998224, 145.0000000000000284 ) ) ;
#8495=FACE_OUTER_BOUND ( 'NONE', #6251, .T. ) ;
#8497=VERTEX_POINT ( 'NONE', #7250 ) ;
#8501=PLANE ( 'NONE',  #7541 ) ;
#8504=LINE ( 'NONE', #7810, #3608 ) ;
#8507=CARTESIAN_POINT ( 'NONE',  ( -4.999999999999998224, 5.000000000000001776, 139.9990000000000236 ) ) ;
#8517=VERTEX_POINT ( 'NONE', #641 ) ;
#8520=CARTESIAN_POINT ( 'NONE',  ( 386.6666666666666288, -15.00000000000000000, 159.8500000000001080 ) ) ;
#8526=ORIENTED_EDGE ( 'NONE', *, *, #60, .T. ) ;
#8532=VECTOR ( 'NONE', #6896, 1000.000000000000000 ) ;
#8539=CYLINDRICAL_SURFACE ( 'NONE', #6330, 2.649999999999985700 ) ;
#8548=AXIS2_PLACEMENT_3D ( 'NONE', #3095, #3264, #5904 ) ;
#8560=DIRECTION ( 'NONE',  ( -0.000000000000000000, 1.000000000000000000, -0.000000000000000000 ) ) ;
#8571=CARTESIAN_POINT ( 'NONE',  ( -30.00000000000000000, -15.00000000000000000, 145.0000000000000284 ) ) ;
#8574=FACE_BOUND ( 'NONE', #5897, .T. ) ;
#8583=PRODUCT ( 'side rail', 'side rail', '', ( #4252 ) ) ;
#8585=EDGE_LOOP ( 'NONE', ( #2689, #8213, #2163, #7782 ) ) ;
#8594=CARTESIAN_POINT ( 'NONE',  ( 136.6666666666666288, -20.00000000000000000, 165.1500000000000625 ) ) ;
#8597=CARTESIAN_POINT ( 'NONE',  ( -4.999999999999998224, -4.999999999999998224, 140.0000000000000000 ) ) ;
#8644=COLOUR_RGB('Light Blue',0.38,0.62,0.78);
#8645=FILL_AREA_STYLE_COLOUR('',#8644);
#8646=FILL_AREA_STYLE('',(#8645));
#8647=SURFACE_STYLE_FILL_AREA(#8646);
#8648=SURFACE_SIDE_STYLE('',(#8647));
#8649=SURFACE_STYLE_USAGE(.BOTH.,#8648);
#8650=PRESENTATION_STYLE_ASSIGNMENT((#8649));
ENDSEC;
END-ISO-10303-21;
